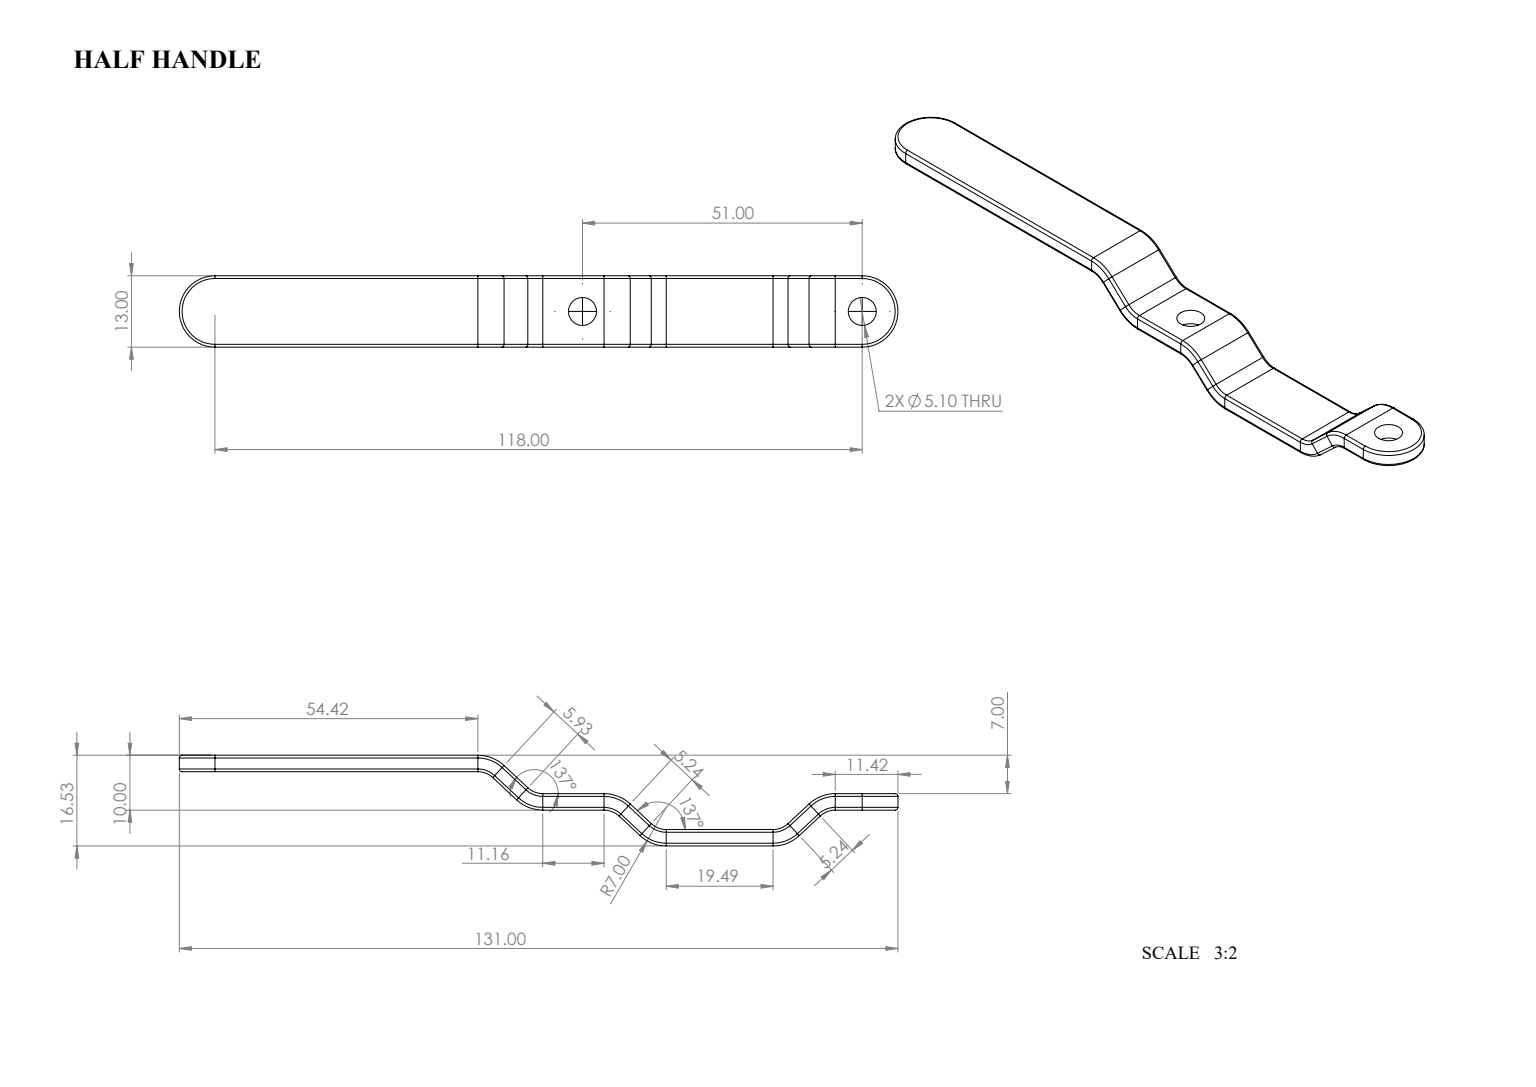
ISO-10303-21;
HEADER;
FILE_DESCRIPTION (('STEP AP214'),
    '1' );
FILE_NAME ('Half Handle.step',
    '2026-10-06T08:09:25',
    ( '' ),
    ( '' ),
    'SwSTEP 2.0',
    'SolidWorks 2021',
    '' );
FILE_SCHEMA (( 'AUTOMOTIVE_DESIGN' ));
ENDSEC;

DATA;
#3=ORIENTED_EDGE ( 'NONE', *, *, #3053, .T. ) ;
#15=CYLINDRICAL_SURFACE ( 'NONE', #19275, 7.000000000000075495 ) ;
#16=FACE_OUTER_BOUND ( 'NONE', #19834, .T. ) ;
#35=ORIENTED_EDGE ( 'NONE', *, *, #12081, .T. ) ;
#44=EDGE_CURVE ( 'NONE', #15578, #10139, #5040, .T. ) ;
#57=TOROIDAL_SURFACE ( 'NONE', #21466, 6.000000000000000000, 0.5000000000000000000 ) ;
#61=ORIENTED_EDGE ( 'NONE', *, *, #623, .T. ) ;
#71=DIRECTION ( 'NONE',  ( -1.000000000000000000, -5.598259082250514647E-17, -3.330669073875432643E-16 ) ) ;
#74=CARTESIAN_POINT ( 'NONE',  ( 119.5756419024615838, -4.500000000000059508, -6.499999999999970690 ) ) ;
#75=AXIS2_PLACEMENT_3D ( 'NONE', #705, #21992, #9988 ) ;
#79=CARTESIAN_POINT ( 'NONE',  ( 2.775557561562891351E-14, 0.000000000000000000, -6.000000000000019540 ) ) ;
#87=ORIENTED_EDGE ( 'NONE', *, *, #1268, .T. ) ;
#102=DIRECTION ( 'NONE',  ( 0.000000000000000000, 0.000000000000000000, 1.000000000000000000 ) ) ;
#108=EDGE_CURVE ( 'NONE', #6044, #8580, #6954, .T. ) ;
#110=DIRECTION ( 'NONE',  ( 3.032184104443271834E-30, 1.000000000000000000, 4.437342591868167759E-31 ) ) ;
#113=DIRECTION ( 'NONE',  ( -0.7313537016191756779, 0.6819983600624930364, -4.478224685260177339E-16 ) ) ;
#125=DIRECTION ( 'NONE',  ( -3.885780586188016830E-16, -4.437342591868156373E-31, 1.000000000000000000 ) ) ;
#147=ORIENTED_EDGE ( 'NONE', *, *, #4920, .T. ) ;
#148=CARTESIAN_POINT ( 'NONE',  ( 119.5756419024615269, -11.00000000000006573, 6.000000000000081712 ) ) ;
#165=FACE_OUTER_BOUND ( 'NONE', #636, .T. ) ;
#169=ADVANCED_FACE ( 'NONE', ( #20745 ), #4609, .T. ) ;
#179=LINE ( 'NONE', #15827, #9133 ) ;
#210=LINE ( 'NONE', #7721, #18126 ) ;
#216=DIRECTION ( 'NONE',  ( 1.000000000000000000, 5.598259082250514647E-17, 3.330669073875432643E-16 ) ) ;
#231=CARTESIAN_POINT ( 'NONE',  ( 54.42435809754113052, -4.000000000000003553, -6.000000000000012434 ) ) ;
#232=LINE ( 'NONE', #4899, #1007 ) ;
#234=DIRECTION ( 'NONE',  ( 0.000000000000000000, 0.000000000000000000, 1.000000000000000000 ) ) ;
#239=DIRECTION ( 'NONE',  ( -1.000000000000000000, 0.000000000000000000, -3.330669073875408978E-16 ) ) ;
#246=ORIENTED_EDGE ( 'NONE', *, *, #14573, .F. ) ;
#248=ADVANCED_FACE ( 'NONE', ( #1437 ), #12950, .T. ) ;
#253=ADVANCED_FACE ( 'NONE', ( #8611 ), #5204, .T. ) ;
#262=LINE ( 'NONE', #18378, #17735 ) ;
#265=CIRCLE ( 'NONE', #18661, 4.500000000000045297 ) ;
#271=ORIENTED_EDGE ( 'NONE', *, *, #15321, .T. ) ;
#273=VERTEX_POINT ( 'NONE', #8728 ) ;
#277=EDGE_LOOP ( 'NONE', ( #6331, #5519, #19401, #7762 ) ) ;
#284=ORIENTED_EDGE ( 'NONE', *, *, #7716, .T. ) ;
#287=CARTESIAN_POINT ( 'NONE',  ( 54.42435809754115894, 2.999999999999947153, 6.000000000000136779 ) ) ;
#291=LINE ( 'NONE', #18180, #3856 ) ;
#299=AXIS2_PLACEMENT_3D ( 'NONE', #21279, #216, #10679 ) ;
#306=EDGE_LOOP ( 'NONE', ( #6785, #17565, #11984, #16573 ) ) ;
#314=ORIENTED_EDGE ( 'NONE', *, *, #20628, .F. ) ;
#315=CARTESIAN_POINT ( 'NONE',  ( 56.34099918003215635, 0.3656768508095153969, -5.999999999999991118 ) ) ;
#317=FACE_OUTER_BOUND ( 'NONE', #6393, .T. ) ;
#324=CARTESIAN_POINT ( 'NONE',  ( 88.75737332930587797, -10.52760560296347947, 6.500000000000075495 ) ) ;
#330=AXIS2_PLACEMENT_3D ( 'NONE', #11225, #18403, #21944 ) ;
#345=VECTOR ( 'NONE', #22191, 1000.000000000000114 ) ;
#349=CARTESIAN_POINT ( 'NONE',  ( 66.26395429947835680, -6.500000000000005329, -6.500000000000081712 ) ) ;
#350=FACE_OUTER_BOUND ( 'NONE', #12361, .T. ) ;
#351=DIRECTION ( 'NONE',  ( -1.000000000000000000, -2.699383410053119644E-30, -3.330669073875432643E-16 ) ) ;
#354=FACE_OUTER_BOUND ( 'NONE', #13443, .T. ) ;
#355=LINE ( 'NONE', #4202, #16056 ) ;
#362=FACE_OUTER_BOUND ( 'NONE', #15798, .T. ) ;
#374=EDGE_LOOP ( 'NONE', ( #13092, #17364, #11552, #11898 ) ) ;
#375=CARTESIAN_POINT ( 'NONE',  ( 108.2426266706972058, -6.527605602963671316, -6.500000000000019540 ) ) ;
#386=AXIS2_PLACEMENT_3D ( 'NONE', #9346, #14745, #22046 ) ;
#397=ORIENTED_EDGE ( 'NONE', *, *, #3887, .T. ) ;
#402=ORIENTED_EDGE ( 'NONE', *, *, #7849, .T. ) ;
#417=ORIENTED_EDGE ( 'NONE', *, *, #17478, .T. ) ;
#430=VECTOR ( 'NONE', #5625, 1000.000000000000114 ) ;
#447=ORIENTED_EDGE ( 'NONE', *, *, #16080, .F. ) ;
#450=DIRECTION ( 'NONE',  ( 3.032184104443272185E-30, 1.000000000000000000, -7.395570986447005381E-32 ) ) ;
#457=DIRECTION ( 'NONE',  ( -3.885780586188016830E-16, -4.437342591868156373E-31, 1.000000000000000000 ) ) ;
#467=CARTESIAN_POINT ( 'NONE',  ( 61.83096495907209089, -4.753799060524588782, 6.500000000000179412 ) ) ;
#468=CARTESIAN_POINT ( 'NONE',  ( 108.2426266706970353, -6.527605602963587828, 6.500000000000199840 ) ) ;
#504=CIRCLE ( 'NONE', #11000, 0.5000000000000033307 ) ;
#519=EDGE_CURVE ( 'NONE', #5606, #14358, #3300, .T. ) ;
#522=VERTEX_POINT ( 'NONE', #22826 ) ;
#542=DIRECTION ( 'NONE',  ( -4.003208021484906984E-16, 0.000000000000000000, 1.000000000000000000 ) ) ;
#550=DIRECTION ( 'NONE',  ( -1.000000000000000000, 7.477632011778292156E-48, -3.885780586188017323E-16 ) ) ;
#552=CLOSED_SHELL ( 'NONE', ( #5998, #12224, #22308, #16919, #14838, #610, #17542, #5814, #9022, #13526, #11262, #22008, #12800, #12847, #7373, #1350, #6364, #15263, #7801, #12373, #8928, #19017, #2140, #3076, #20370, #13608, #253, #7841, #18717, #10097, #22749, #10522, #2281, #5956, #13001, #8303, #15121, #2768, #13653, #19566, #15676, #20490, #22930, #18573, #22774, #6659, #16164, #8294, #8684, #5013, #2022, #6644, #17118, #6392, #7909, #19774, #10655, #21216, #20630, #3506, #12830, #8059, #21456, #15577, #6060, #7869, #10599, #15845, #17708, #12378, #6678, #19804, #5540, #19247, #5780, #21642, #16295, #19370, #13968, #12259, #9663, #1243, #17730, #12097, #1896, #687, #20297, #21117, #20746, #4689, #12071, #17436, #7470, #15967, #6389, #3205, #13846, #14982, #16297, #15524, #6855, #17451, #21619, #3605, #12668, #248, #4912, #22621, #14523, #15294, #7422, #169, #14422, #14548 ) ) ;
#568=SHAPE_REPRESENTATION_RELATIONSHIP ( 'NONE' , 'NONE' ,  #15574, #22653 ) ;
#572=EDGE_LOOP ( 'NONE', ( #5727, #7824, #20773, #18885 ) ) ;
#573=CARTESIAN_POINT ( 'NONE',  ( 115.1426525620552894, -6.246200939475421876, 6.000000000000158096 ) ) ;
#585=CARTESIAN_POINT ( 'NONE',  ( 58.85734743794737511, 0.7537990605245015185, -6.499999999999895195 ) ) ;
#589=DIRECTION ( 'NONE',  ( 0.6819983600624954789, 0.7313537016191733464, 7.771699578536739269E-16 ) ) ;
#590=CARTESIAN_POINT ( 'NONE',  ( 66.26395429947839943, -7.000000000000006217, -6.499999999999999112 ) ) ;
#593=VECTOR ( 'NONE', #7277, 1000.000000000000000 ) ;
#601=DIRECTION ( 'NONE',  ( -1.000000000000000000, -2.699383410053119644E-30, -3.330669073875432643E-16 ) ) ;
#610=ADVANCED_FACE ( 'NONE', ( #4927 ), #12094, .F. ) ;
#623=EDGE_CURVE ( 'NONE', #15916, #8376, #10912, .T. ) ;
#626=EDGE_CURVE ( 'NONE', #2822, #21618, #7403, .T. ) ;
#636=EDGE_LOOP ( 'NONE', ( #3298, #20514, #22207, #18614 ) ) ;
#669=DIRECTION ( 'NONE',  ( 1.000000000000000000, 2.699383410053119644E-30, 3.330669073875432643E-16 ) ) ;
#677=DIRECTION ( 'NONE',  ( 3.032184104443272185E-30, 1.000000000000000000, -7.395570986447005381E-32 ) ) ;
#678=AXIS2_PLACEMENT_3D ( 'NONE', #13630, #15379, #15731 ) ;
#683=SURFACE_SIDE_STYLE ('',( #9387 ) ) ;
#687=ADVANCED_FACE ( 'NONE', ( #21534 ), #20120, .T. ) ;
#693=DIRECTION ( 'NONE',  ( 0.6819983600624958120, 0.7313537016191731244, 7.771699578536736311E-16 ) ) ;
#694=LINE ( 'NONE', #5870, #6828 ) ;
#700=VERTEX_POINT ( 'NONE', #19396 ) ;
#701=LINE ( 'NONE', #13282, #21174 ) ;
#704=ORIENTED_EDGE ( 'NONE', *, *, #6611, .T. ) ;
#705=CARTESIAN_POINT ( 'NONE',  ( 54.42435809754115894, 2.499999999999946709, 6.000000000000136779 ) ) ;
#712=( GEOMETRIC_REPRESENTATION_CONTEXT ( 3 ) GLOBAL_UNCERTAINTY_ASSIGNED_CONTEXT ( ( #16830 ) ) GLOBAL_UNIT_ASSIGNED_CONTEXT ( ( #5192, #21975, #2204 ) ) REPRESENTATION_CONTEXT ( 'NONE', 'WORKASPACE' ) );
#717=ORIENTED_EDGE ( 'NONE', *, *, #22216, .T. ) ;
#720=DIRECTION ( 'NONE',  ( 1.000000000000000000, 2.699383410053119644E-30, 3.330669073875432643E-16 ) ) ;
#730=AXIS2_PLACEMENT_3D ( 'NONE', #8897, #17709, #6781 ) ;
#740=EDGE_LOOP ( 'NONE', ( #2269, #18796, #14103, #12386 ) ) ;
#746=VERTEX_POINT ( 'NONE', #5056 ) ;
#763=LINE ( 'NONE', #20873, #11220 ) ;
#766=EDGE_CURVE ( 'NONE', #11435, #5256, #21184, .T. ) ;
#773=CIRCLE ( 'NONE', #10164, 0.5000000000000038858 ) ;
#788=EDGE_CURVE ( 'NONE', #15578, #6044, #1862, .T. ) ;
#795=CARTESIAN_POINT ( 'NONE',  ( 6.500000000000227374, 2.500000000000196287, 6.000000000000213163 ) ) ;
#797=FILL_AREA_STYLE ('',( #2314 ) ) ;
#801=ORIENTED_EDGE ( 'NONE', *, *, #10616, .F. ) ;
#802=AXIS2_PLACEMENT_3D ( 'NONE', #12809, #5296, #239 ) ;
#816=CARTESIAN_POINT ( 'NONE',  ( 6.500000000000366818, 2.500000000000196287, 6.500000000000123457 ) ) ;
#821=AXIS2_PLACEMENT_3D ( 'NONE', #3851, #21982, #16435 ) ;
#831=CIRCLE ( 'NONE', #9848, 4.000000000000045297 ) ;
#843=DIRECTION ( 'NONE',  ( 1.000000000000000000, 0.000000000000000000, 4.336808689941968432E-16 ) ) ;
#861=ORIENTED_EDGE ( 'NONE', *, *, #20330, .T. ) ;
#868=CARTESIAN_POINT ( 'NONE',  ( 88.75737332930597745, -13.52760560296348302, 6.500000000000103029 ) ) ;
#934=DIRECTION ( 'NONE',  ( 0.000000000000000000, 0.000000000000000000, 1.000000000000000000 ) ) ;
#935=DIRECTION ( 'NONE',  ( -0.7313537016191756779, 0.6819983600624930364, -4.478224685260177339E-16 ) ) ;
#941=DIRECTION ( 'NONE',  ( -1.000000000000000000, -2.699383410053119644E-30, -3.330669073875432643E-16 ) ) ;
#961=DIRECTION ( 'NONE',  ( -1.000000000000000000, -2.699383410053119644E-30, -3.330669073875432643E-16 ) ) ;
#973=DIRECTION ( 'NONE',  ( -1.000000000000000000, -2.699383410053119644E-30, -3.330669073875432643E-16 ) ) ;
#979=EDGE_CURVE ( 'NONE', #11432, #5256, #232, .T. ) ;
#982=ORIENTED_EDGE ( 'NONE', *, *, #6089, .T. ) ;
#1000=DIRECTION ( 'NONE',  ( 3.885780586188016830E-16, 4.437342591868156373E-31, -1.000000000000000000 ) ) ;
#1007=VECTOR ( 'NONE', #1279, 1000.000000000000000 ) ;
#1053=AXIS2_PLACEMENT_3D ( 'NONE', #9891, #961, #12100 ) ;
#1060=CARTESIAN_POINT ( 'NONE',  ( 119.5756419024615838, -6.500000000000061284, -5.999999999999984901 ) ) ;
#1064=LINE ( 'NONE', #10212, #4061 ) ;
#1070=AXIS2_PLACEMENT_3D ( 'NONE', #12709, #1992, #1876 ) ;
#1073=ORIENTED_EDGE ( 'NONE', *, *, #6663, .T. ) ;
#1075=CARTESIAN_POINT ( 'NONE',  ( 59.19834661797866460, 1.119475911334100182, 6.500000000000130562 ) ) ;
#1086=EDGE_CURVE ( 'NONE', #16898, #10112, #2677, .T. ) ;
#1091=AXIS2_PLACEMENT_3D ( 'NONE', #18092, #10900, #9266 ) ;
#1096=ORIENTED_EDGE ( 'NONE', *, *, #3338, .T. ) ;
#1106=CARTESIAN_POINT ( 'NONE',  ( 85.68838070902455684, -9.818697260249752645, 6.000000000000136779 ) ) ;
#1110=EDGE_CURVE ( 'NONE', #11343, #15739, #11136, .T. ) ;
#1111=DIRECTION ( 'NONE',  ( 3.032184104443272185E-30, 1.000000000000000000, -7.395570986447005381E-32 ) ) ;
#1116=DIRECTION ( 'NONE',  ( -0.7313537016191773432, 0.6819983600624913711, 1.628001950178159721E-16 ) ) ;
#1118=EDGE_CURVE ( 'NONE', #13735, #11435, #20927, .T. ) ;
#1122=DIRECTION ( 'NONE',  ( 3.885780586188016830E-16, 4.437342591868156373E-31, -1.000000000000000000 ) ) ;
#1126=EDGE_LOOP ( 'NONE', ( #14306, #4368, #8291, #9544 ) ) ;
#1128=ORIENTED_EDGE ( 'NONE', *, *, #17861, .F. ) ;
#1138=DIRECTION ( 'NONE',  ( -3.885780586188016830E-16, -4.437342591868156373E-31, 1.000000000000000000 ) ) ;
#1145=AXIS2_PLACEMENT_3D ( 'NONE', #5595, #16499, #9229 ) ;
#1156=ORIENTED_EDGE ( 'NONE', *, *, #626, .F. ) ;
#1157=ORIENTED_EDGE ( 'NONE', *, *, #788, .T. ) ;
#1159=DIRECTION ( 'NONE',  ( -0.6819983600625064701, -0.7313537016191632434, 0.000000000000000000 ) ) ;
#1160=ORIENTED_EDGE ( 'NONE', *, *, #10930, .T. ) ;
#1166=CARTESIAN_POINT ( 'NONE',  ( 113.0166151911346617, -11.64708151429780258, 6.500000000000110134 ) ) ;
#1170=DIRECTION ( 'NONE',  ( 1.000000000000000000, 2.699383410053119644E-30, 3.330669073875432643E-16 ) ) ;
#1173=EDGE_CURVE ( 'NONE', #746, #20880, #10395, .T. ) ;
#1210=EDGE_CURVE ( 'NONE', #23117, #22529, #21623, .T. ) ;
#1211=EDGE_LOOP ( 'NONE', ( #10687, #3, #21937, #717 ) ) ;
#1231=FACE_OUTER_BOUND ( 'NONE', #3457, .T. ) ;
#1243=ADVANCED_FACE ( 'NONE', ( #18852 ), #10767, .T. ) ;
#1244=CIRCLE ( 'NONE', #16614, 0.4999999999999997224 ) ;
#1253=DIRECTION ( 'NONE',  ( -0.7313537016191753448, -0.6819983600624934805, -1.628001950178158981E-16 ) ) ;
#1254=DIRECTION ( 'NONE',  ( 3.032184104443271834E-30, 1.000000000000000000, 4.437342591868167759E-31 ) ) ;
#1268=EDGE_CURVE ( 'NONE', #6421, #12056, #9925, .T. ) ;
#1269=EDGE_LOOP ( 'NONE', ( #6367, #10826, #1697, #13479 ) ) ;
#1271=EDGE_CURVE ( 'NONE', #11689, #5606, #19039, .T. ) ;
#1279=DIRECTION ( 'NONE',  ( -0.7313537016191735685, 0.6819983600624951459, -3.923113172947598083E-16 ) ) ;
#1288=DIRECTION ( 'NONE',  ( 0.000000000000000000, 0.000000000000000000, 1.000000000000000000 ) ) ;
#1294=AXIS2_PLACEMENT_3D ( 'NONE', #19329, #22516, #6859 ) ;
#1303=LINE ( 'NONE', #8350, #11618 ) ;
#1311=VECTOR ( 'NONE', #6045, 1000.000000000000114 ) ;
#1331=EDGE_LOOP ( 'NONE', ( #20654, #22644, #11760, #18194 ) ) ;
#1332=CARTESIAN_POINT ( 'NONE',  ( 88.75737332930594903, -6.527605602963476805, 6.500000000000151879 ) ) ;
#1335=CARTESIAN_POINT ( 'NONE',  ( 88.75737332930594903, -13.02760560296348302, 6.000000000000130562 ) ) ;
#1350=ADVANCED_FACE ( 'NONE', ( #7920 ), #4263, .T. ) ;
#1369=PLANE ( 'NONE',  #20431 ) ;
#1378=ORIENTED_EDGE ( 'NONE', *, *, #10707, .F. ) ;
#1389=CARTESIAN_POINT ( 'NONE',  ( 119.5756419024615838, -11.00000000000006573, -6.500000000000075495 ) ) ;
#1391=DIRECTION ( 'NONE',  ( 0.6819983600624981435, -0.7313537016191709039, 0.000000000000000000 ) ) ;
#1409=ORIENTED_EDGE ( 'NONE', *, *, #4321, .T. ) ;
#1421=DIRECTION ( 'NONE',  ( -3.885780586188016830E-16, -4.437342591868156373E-31, 1.000000000000000000 ) ) ;
#1427=ORIENTED_EDGE ( 'NONE', *, *, #5079, .T. ) ;
#1436=CARTESIAN_POINT ( 'NONE',  ( 58.85734743794750301, 0.7537990605245015185, -5.999999999999880096 ) ) ;
#1437=FACE_OUTER_BOUND ( 'NONE', #5827, .T. ) ;
#1440=CARTESIAN_POINT ( 'NONE',  ( 80.49335071782263640, -7.708908342713538531, 6.500000000000033751 ) ) ;
#1453=DIRECTION ( 'NONE',  ( 3.885780586188016830E-16, 4.437342591868156373E-31, -1.000000000000000000 ) ) ;
#1457=ORIENTED_EDGE ( 'NONE', *, *, #11127, .F. ) ;
#1469=ORIENTED_EDGE ( 'NONE', *, *, #108, .F. ) ;
#1474=PLANE ( 'NONE',  #8000 ) ;
#1495=VERTEX_POINT ( 'NONE', #1440 ) ;
#1511=DIRECTION ( 'NONE',  ( 0.7313537016191745677, 0.6819983600624940356, 1.072890437865584285E-16 ) ) ;
#1518=ORIENTED_EDGE ( 'NONE', *, *, #20201, .T. ) ;
#1522=EDGE_CURVE ( 'NONE', #22506, #18271, #8616, .T. ) ;
#1528=EDGE_CURVE ( 'NONE', #11543, #15515, #17880, .T. ) ;
#1529=DIRECTION ( 'NONE',  ( 0.6819983600625074693, -0.7313537016191621332, 1.110084618464482116E-16 ) ) ;
#1549=CIRCLE ( 'NONE', #7564, 0.5000000000000038858 ) ;
#1553=CARTESIAN_POINT ( 'NONE',  ( 82.19834661797897013, -5.880524088665628923, 6.500000000000151879 ) ) ;
#1566=AXIS2_PLACEMENT_3D ( 'NONE', #17345, #1253, #8430 ) ;
#1567=DIRECTION ( 'NONE',  ( 3.885780586188016830E-16, 4.437342591868156373E-31, -1.000000000000000000 ) ) ;
#1568=PLANE ( 'NONE',  #3642 ) ;
#1573=ORIENTED_EDGE ( 'NONE', *, *, #2157, .F. ) ;
#1578=AXIS2_PLACEMENT_3D ( 'NONE', #16932, #6256, #843 ) ;
#1587=CARTESIAN_POINT ( 'NONE',  ( 77.42435809754145737, -6.499999999999811706, -6.499999999999984901 ) ) ;
#1604=CIRCLE ( 'NONE', #3842, 0.5000000000000038858 ) ;
#1609=PRODUCT_DEFINITION_SHAPE ( 'NONE', 'NONE',  #17672 ) ;
#1610=ORIENTED_EDGE ( 'NONE', *, *, #10575, .T. ) ;
#1611=CARTESIAN_POINT ( 'NONE',  ( 80.15235153779146060, -8.074585193523137860, 6.000000000000109246 ) ) ;
#1614=CARTESIAN_POINT ( 'NONE',  ( 77.42435809754135789, -10.99999999999981526, 6.500000000000123457 ) ) ;
#1617=LINE ( 'NONE', #19377, #10224 ) ;
#1621=VECTOR ( 'NONE', #16837, 1000.000000000000000 ) ;
#1634=AXIS2_PLACEMENT_3D ( 'NONE', #16389, #23134, #5714 ) ;
#1660=AXIS2_PLACEMENT_3D ( 'NONE', #8212, #6447, #1159 ) ;
#1667=EDGE_LOOP ( 'NONE', ( #61, #23206, #12396, #397 ) ) ;
#1668=ORIENTED_EDGE ( 'NONE', *, *, #16268, .F. ) ;
#1676=DIRECTION ( 'NONE',  ( -3.241725282392603095E-30, -1.000000000000000000, 2.218671295934100958E-31 ) ) ;
#1697=ORIENTED_EDGE ( 'NONE', *, *, #2183, .F. ) ;
#1701=EDGE_LOOP ( 'NONE', ( #3380, #9857, #18964, #1457 ) ) ;
#1709=DIRECTION ( 'NONE',  ( 3.330669073875432643E-16, 4.437342591868153746E-31, -1.000000000000000000 ) ) ;
#1723=EDGE_CURVE ( 'NONE', #19565, #9737, #4469, .T. ) ;
#1724=CARTESIAN_POINT ( 'NONE',  ( 73.50000000000116529, -13.52760560296348302, 3.469446951953614189E-14 ) ) ;
#1739=CYLINDRICAL_SURFACE ( 'NONE', #10098, 0.4999999999999978351 ) ;
#1758=AXIS2_PLACEMENT_3D ( 'NONE', #10952, #18261, #3785 ) ;
#1769=VECTOR ( 'NONE', #973, 1000.000000000000000 ) ;
#1795=DIRECTION ( 'NONE',  ( 0.000000000000000000, 0.000000000000000000, 1.000000000000000000 ) ) ;
#1798=DIRECTION ( 'NONE',  ( -0.7313537016191746787, -0.6819983600624940356, -1.072890437865584285E-16 ) ) ;
#1799=DIRECTION ( 'NONE',  ( 3.885780586188016830E-16, 4.437342591868156373E-31, -1.000000000000000000 ) ) ;
#1812=ORIENTED_EDGE ( 'NONE', *, *, #16958, .F. ) ;
#1814=AXIS2_PLACEMENT_3D ( 'NONE', #21549, #12588, #18016 ) ;
#1821=LINE ( 'NONE', #23253, #8978 ) ;
#1822=CARTESIAN_POINT ( 'NONE',  ( 73.50000000000116529, -6.999999999999811706, -2.549999999999999822 ) ) ;
#1827=ORIENTED_EDGE ( 'NONE', *, *, #20596, .F. ) ;
#1828=CIRCLE ( 'NONE', #22491, 0.5000000000000038858 ) ;
#1829=DIRECTION ( 'NONE',  ( 3.885780586188016830E-16, 4.437342591868156373E-31, -1.000000000000000000 ) ) ;
#1839=CYLINDRICAL_SURFACE ( 'NONE', #20758, 4.000000000000045297 ) ;
#1860=AXIS2_PLACEMENT_3D ( 'NONE', #19707, #7012, #12163 ) ;
#1862=LINE ( 'NONE', #9046, #20910 ) ;
#1865=ORIENTED_EDGE ( 'NONE', *, *, #2806, .F. ) ;
#1871=DIRECTION ( 'NONE',  ( 1.000000000000000000, 2.699383410053119644E-30, 3.330669073875432643E-16 ) ) ;
#1876=DIRECTION ( 'NONE',  ( 0.000000000000000000, 0.000000000000000000, 1.000000000000000000 ) ) ;
#1889=VECTOR ( 'NONE', #3441, 1000.000000000000000 ) ;
#1892=EDGE_CURVE ( 'NONE', #4169, #16118, #8245, .T. ) ;
#1894=FACE_OUTER_BOUND ( 'NONE', #9998, .T. ) ;
#1896=ADVANCED_FACE ( 'NONE', ( #22591 ), #19404, .T. ) ;
#1908=AXIS2_PLACEMENT_3D ( 'NONE', #16553, #16096, #10814 ) ;
#1909=AXIS2_PLACEMENT_3D ( 'NONE', #12173, #5123, #19476 ) ;
#1912=EDGE_CURVE ( 'NONE', #22610, #5349, #17519, .T. ) ;
#1918=ORIENTED_EDGE ( 'NONE', *, *, #12888, .F. ) ;
#1920=DIRECTION ( 'NONE',  ( 1.000000000000000000, 2.699383410053119644E-30, 3.330669073875432643E-16 ) ) ;
#1928=DIRECTION ( 'NONE',  ( -1.000000000000000000, -2.699383410053119644E-30, -3.330669073875432643E-16 ) ) ;
#1929=CARTESIAN_POINT ( 'NONE',  ( 54.42435809754115894, 0.4999999999999449329, -5.999999999999950262 ) ) ;
#1934=ORIENTED_EDGE ( 'NONE', *, *, #20891, .F. ) ;
#1946=FACE_OUTER_BOUND ( 'NONE', #3552, .T. ) ;
#1947=CARTESIAN_POINT ( 'NONE',  ( 108.2426266706970353, -6.527605602963587828, 6.500000000000199840 ) ) ;
#1949=DIRECTION ( 'NONE',  ( 3.885780586188016830E-16, 4.437342591868156373E-31, -1.000000000000000000 ) ) ;
#1950=CIRCLE ( 'NONE', #6480, 6.500000000000075495 ) ;
#1955=CIRCLE ( 'NONE', #8719, 6.500000000000075495 ) ;
#1956=CARTESIAN_POINT ( 'NONE',  ( 88.75737332930596324, -13.52760560296348302, -6.499999999999964473 ) ) ;
#1967=CIRCLE ( 'NONE', #15113, 0.5000000000000038858 ) ;
#1968=ORIENTED_EDGE ( 'NONE', *, *, #20201, .F. ) ;
#1983=CARTESIAN_POINT ( 'NONE',  ( 119.5756419024615553, -11.00000000000006573, 6.500000000000012434 ) ) ;
#1992=DIRECTION ( 'NONE',  ( -1.000000000000000000, -2.699383410053119644E-30, -3.330669073875432643E-16 ) ) ;
#2004=DIRECTION ( 'NONE',  ( -1.000000000000000000, 1.773272886554051558E-14, -3.854941057726199147E-16 ) ) ;
#2015=DIRECTION ( 'NONE',  ( -1.000000000000000000, 1.847414967615758933E-47, -3.885780586188017323E-16 ) ) ;
#2022=ADVANCED_FACE ( 'NONE', ( #16 ), #14344, .T. ) ;
#2040=EDGE_CURVE ( 'NONE', #10112, #11689, #17882, .T. ) ;
#2042=DIRECTION ( 'NONE',  ( -1.000000000000000000, -2.699383410053119644E-30, -3.330669073875432643E-16 ) ) ;
#2062=EDGE_CURVE ( 'NONE', #15653, #23176, #8567, .T. ) ;
#2078=CARTESIAN_POINT ( 'NONE',  ( 61.48996577904087957, -5.119475911334187224, -5.999999999999943157 ) ) ;
#2091=DIRECTION ( 'NONE',  ( -1.000000000000000000, 0.000000000000000000, -4.336808689941968432E-16 ) ) ;
#2106=CARTESIAN_POINT ( 'NONE',  ( 86.02937988905577527, -11.02760560296348125, -5.999999999999991118 ) ) ;
#2115=ORIENTED_EDGE ( 'NONE', *, *, #17411, .T. ) ;
#2129=LINE ( 'NONE', #14497, #20800 ) ;
#2140=ADVANCED_FACE ( 'NONE', ( #16905 ), #2223, .T. ) ;
#2142=ORIENTED_EDGE ( 'NONE', *, *, #9809, .F. ) ;
#2145=ORIENTED_EDGE ( 'NONE', *, *, #12997, .F. ) ;
#2155=CARTESIAN_POINT ( 'NONE',  ( 110.9706201109470811, -9.453020409440348715, -5.999999999999956479 ) ) ;
#2157=EDGE_CURVE ( 'NONE', #746, #9743, #355, .T. ) ;
#2165=DIRECTION ( 'NONE',  ( 0.000000000000000000, 0.000000000000000000, 1.000000000000000000 ) ) ;
#2171=AXIS2_PLACEMENT_3D ( 'NONE', #12179, #17600, #23264 ) ;
#2172=EDGE_LOOP ( 'NONE', ( #20562, #16691, #3291, #6613 ) ) ;
#2174=FACE_OUTER_BOUND ( 'NONE', #14632, .T. ) ;
#2178=ORIENTED_EDGE ( 'NONE', *, *, #5139, .F. ) ;
#2183=EDGE_CURVE ( 'NONE', #522, #22680, #12297, .T. ) ;
#2188=DIRECTION ( 'NONE',  ( 1.000000000000000000, 1.599800538956372742E-14, 3.854941057726199147E-16 ) ) ;
#2197=CYLINDRICAL_SURFACE ( 'NONE', #13937, 7.000000000000075495 ) ;
#2204=( NAMED_UNIT ( * ) SI_UNIT ( $, .STERADIAN. ) SOLID_ANGLE_UNIT ( ) );
#2209=EDGE_CURVE ( 'NONE', #18644, #14732, #20963, .T. ) ;
#2213=DIRECTION ( 'NONE',  ( -0.7313537016191794526, -0.6819983600624889286, -4.403559511741029625E-16 ) ) ;
#2215=ORIENTED_EDGE ( 'NONE', *, *, #1528, .T. ) ;
#2223=PLANE ( 'NONE',  #22844 ) ;
#2226=CARTESIAN_POINT ( 'NONE',  ( 77.42435809754137210, -6.999999999999811706, 6.500000000000081712 ) ) ;
#2230=PLANE ( 'NONE',  #10685 ) ;
#2231=CARTESIAN_POINT ( 'NONE',  ( 119.9981234580896796, -4.453056000818161664, 6.000000000000123457 ) ) ;
#2235=EDGE_CURVE ( 'NONE', #19565, #12056, #7444, .T. ) ;
#2252=DIRECTION ( 'NONE',  ( -0.6819983600624998088, -0.7313537016191693496, 0.000000000000000000 ) ) ;
#2253=DIRECTION ( 'NONE',  ( 3.241725282392603095E-30, 1.000000000000000000, -2.218671295934100958E-31 ) ) ;
#2256=FILL_AREA_STYLE_COLOUR ( '', #4776 ) ;
#2261=EDGE_CURVE ( 'NONE', #4634, #9218, #7087, .T. ) ;
#2265=ORIENTED_EDGE ( 'NONE', *, *, #12537, .T. ) ;
#2269=ORIENTED_EDGE ( 'NONE', *, *, #8952, .T. ) ;
#2273=EDGE_LOOP ( 'NONE', ( #2521, #9741, #12678, #4333 ) ) ;
#2274=ORIENTED_EDGE ( 'NONE', *, *, #13394, .T. ) ;
#2281=ADVANCED_FACE ( 'NONE', ( #22568 ), #4903, .T. ) ;
#2297=CIRCLE ( 'NONE', #75, 0.5000000000000038858 ) ;
#2298=VECTOR ( 'NONE', #19851, 1000.000000000000000 ) ;
#2314=FILL_AREA_STYLE_COLOUR ( '', #14588 ) ;
#2331=CARTESIAN_POINT ( 'NONE',  ( 108.2426266706970779, -6.527605602963587828, 6.000000000000109246 ) ) ;
#2332=AXIS2_PLACEMENT_3D ( 'NONE', #5854, #16756, #9373 ) ;
#2336=CARTESIAN_POINT ( 'NONE',  ( 109.3164911904586916, -11.67918431276163105, -6.000000000000060396 ) ) ;
#2344=CARTESIAN_POINT ( 'NONE',  ( 116.8476484622115805, -8.074585193523331483, -5.999999999999956479 ) ) ;
#2369=CARTESIAN_POINT ( 'NONE',  ( 57.49335071782248008, -0.7089083427137543580, 6.500000000000088818 ) ) ;
#2381=AXIS2_PLACEMENT_3D ( 'NONE', #1956, #9154, #16314 ) ;
#2386=EDGE_LOOP ( 'NONE', ( #18996, #18444, #16291, #5485 ) ) ;
#2389=AXIS2_PLACEMENT_3D ( 'NONE', #22561, #4553, #2801 ) ;
#2405=AXIS2_PLACEMENT_3D ( 'NONE', #5125, #12286, #12409 ) ;
#2416=DIRECTION ( 'NONE',  ( -0.7313537016191734574, 0.6819983600624954789, -3.733258675956565293E-18 ) ) ;
#2419=CIRCLE ( 'NONE', #9935, 0.5000000000000038858 ) ;
#2435=CARTESIAN_POINT ( 'NONE',  ( 108.2426266706970637, -11.02760560296359138, 5.999999999999984901 ) ) ;
#2451=DIRECTION ( 'NONE',  ( -3.885780586188016830E-16, -4.437342591868156373E-31, 1.000000000000000000 ) ) ;
#2458=DIRECTION ( 'NONE',  ( 3.885780586188016830E-16, 4.437342591868156373E-31, -1.000000000000000000 ) ) ;
#2462=ORIENTED_EDGE ( 'NONE', *, *, #21922, .T. ) ;
#2464=ORIENTED_EDGE ( 'NONE', *, *, #5341, .T. ) ;
#2481=CARTESIAN_POINT ( 'NONE',  ( 124.5000000000019469, -6.500000000000061284, 4.857225732735059864E-14 ) ) ;
#2484=EDGE_CURVE ( 'NONE', #15515, #7123, #21845, .T. ) ;
#2486=LINE ( 'NONE', #20503, #13438 ) ;
#2487=CARTESIAN_POINT ( 'NONE',  ( 66.26395429947835680, -4.500000000000003553, -6.500000000000081712 ) ) ;
#2489=ORIENTED_EDGE ( 'NONE', *, *, #5645, .F. ) ;
#2490=TOROIDAL_SURFACE ( 'NONE', #8901, 6.500000000000000888, 0.5000000000000000000 ) ;
#2492=EDGE_LOOP ( 'NONE', ( #35, #15607, #5667, #17989 ) ) ;
#2493=UNCERTAINTY_MEASURE_WITH_UNIT (LENGTH_MEASURE( 1.000000000000000082E-05 ), #11423, 'distance_accuracy_value', 'NONE');
#2521=ORIENTED_EDGE ( 'NONE', *, *, #13323, .T. ) ;
#2525=CIRCLE ( 'NONE', #7048, 0.4999999999999984457 ) ;
#2531=DIRECTION ( 'NONE',  ( 0.6819983600624981435, -0.7313537016191709039, 0.000000000000000000 ) ) ;
#2538=AXIS2_PLACEMENT_3D ( 'NONE', #2743, #18987, #23079 ) ;
#2552=ORIENTED_EDGE ( 'NONE', *, *, #13276, .T. ) ;
#2567=DIRECTION ( 'NONE',  ( -1.000000000000000000, -2.699383410053119644E-30, -3.330669073875432643E-16 ) ) ;
#2572=DIRECTION ( 'NONE',  ( -3.032184104443272185E-30, -1.000000000000000000, 7.395570986447005381E-32 ) ) ;
#2576=CYLINDRICAL_SURFACE ( 'NONE', #6610, 0.5000000000000038858 ) ;
#2582=CIRCLE ( 'NONE', #19501, 4.000000000000045297 ) ;
#2593=EDGE_CURVE ( 'NONE', #16059, #19782, #2582, .T. ) ;
#2595=AXIS2_PLACEMENT_3D ( 'NONE', #10540, #18195, #9242 ) ;
#2610=ORIENTED_EDGE ( 'NONE', *, *, #15468, .F. ) ;
#2621=CARTESIAN_POINT ( 'NONE',  ( 119.5756419024614559, 2.499999999999974243, -5.999999999999963585 ) ) ;
#2628=APPLICATION_CONTEXT ( 'automotive_design' ) ;
#2639=CYLINDRICAL_SURFACE ( 'NONE', #9314, 7.000000000000075495 ) ;
#2640=EDGE_CURVE ( 'NONE', #23176, #18021, #6653, .T. ) ;
#2641=ORIENTED_EDGE ( 'NONE', *, *, #10946, .T. ) ;
#2643=EDGE_LOOP ( 'NONE', ( #9016, #7011, #20838, #17686 ) ) ;
#2653=CYLINDRICAL_SURFACE ( 'NONE', #7597, 0.4999999999999987232 ) ;
#2659=CARTESIAN_POINT ( 'NONE',  ( 119.5756419024615411, -7.000000000000006217, 6.000000000000095923 ) ) ;
#2665=EDGE_LOOP ( 'NONE', ( #9213, #15572, #3033, #14858 ) ) ;
#2673=DIRECTION ( 'NONE',  ( -0.7313537016191730133, 0.6819983600624957010, -5.924440990721418971E-17 ) ) ;
#2677=LINE ( 'NONE', #11614, #7400 ) ;
#2684=FACE_OUTER_BOUND ( 'NONE', #22293, .T. ) ;
#2688=CARTESIAN_POINT ( 'NONE',  ( 80.49335071782266482, -7.708908342713566064, -6.500000000000047073 ) ) ;
#2697=AXIS2_PLACEMENT_3D ( 'NONE', #18422, #11347, #18538 ) ;
#2705=FACE_OUTER_BOUND ( 'NONE', #15944, .T. ) ;
#2717=CIRCLE ( 'NONE', #5358, 6.000000000000047962 ) ;
#2721=ORIENTED_EDGE ( 'NONE', *, *, #5530, .F. ) ;
#2724=ORIENTED_EDGE ( 'NONE', *, *, #14425, .F. ) ;
#2726=ORIENTED_EDGE ( 'NONE', *, *, #22779, .F. ) ;
#2728=ORIENTED_EDGE ( 'NONE', *, *, #8529, .T. ) ;
#2734=DIRECTION ( 'NONE',  ( -1.000000000000000000, 1.847414967615758933E-47, -3.885780586188017323E-16 ) ) ;
#2737=DIRECTION ( 'NONE',  ( 0.000000000000000000, 0.000000000000000000, -1.000000000000000000 ) ) ;
#2743=CARTESIAN_POINT ( 'NONE',  ( 108.2426266706970637, -13.52760560296348302, 6.500000000000019540 ) ) ;
#2765=APPLICATION_CONTEXT ( 'automotive_design' ) ;
#2766=ORIENTED_EDGE ( 'NONE', *, *, #21500, .T. ) ;
#2768=ADVANCED_FACE ( 'NONE', ( #6428 ), #15115, .T. ) ;
#2786=EDGE_CURVE ( 'NONE', #17843, #3270, #1821, .T. ) ;
#2787=ORIENTED_EDGE ( 'NONE', *, *, #9230, .T. ) ;
#2792=ORIENTED_EDGE ( 'NONE', *, *, #16542, .T. ) ;
#2796=ORIENTED_EDGE ( 'NONE', *, *, #44, .T. ) ;
#2801=DIRECTION ( 'NONE',  ( 1.000000000000000000, -7.477632011778619108E-48, 3.885780586188017323E-16 ) ) ;
#2804=DIRECTION ( 'NONE',  ( -1.000000000000000000, -2.699383410053119644E-30, -3.330669073875432643E-16 ) ) ;
#2806=EDGE_CURVE ( 'NONE', #700, #9743, #12332, .T. ) ;
#2816=AXIS2_PLACEMENT_3D ( 'NONE', #19426, #3327, #12013 ) ;
#2817=LINE ( 'NONE', #2688, #3872 ) ;
#2821=ORIENTED_EDGE ( 'NONE', *, *, #2786, .F. ) ;
#2822=VERTEX_POINT ( 'NONE', #1587 ) ;
#2826=VERTEX_POINT ( 'NONE', #74 ) ;
#2829=EDGE_CURVE ( 'NONE', #6497, #19367, #17467, .T. ) ;
#2845=ORIENTED_EDGE ( 'NONE', *, *, #6203, .F. ) ;
#2853=EDGE_LOOP ( 'NONE', ( #19452, #5309, #11785, #6845 ) ) ;
#2855=DIRECTION ( 'NONE',  ( -0.7313537016191773432, 0.6819983600624913711, 1.628001950178159721E-16 ) ) ;
#2889=CARTESIAN_POINT ( 'NONE',  ( 77.42435809754135789, -10.99999999999981526, 6.500000000000123457 ) ) ;
#2891=DIRECTION ( 'NONE',  ( 0.6819983600625060260, 0.7313537016191635765, 6.106365041599011361E-16 ) ) ;
#2895=DIRECTION ( 'NONE',  ( -1.000000000000000000, 1.847414967615758933E-47, -3.885780586188017323E-16 ) ) ;
#2899=VECTOR ( 'NONE', #6721, 1000.000000000000000 ) ;
#2907=VERTEX_POINT ( 'NONE', #21373 ) ;
#2910=ORIENTED_EDGE ( 'NONE', *, *, #4920, .F. ) ;
#2921=LINE ( 'NONE', #1166, #19297 ) ;
#2922=DIRECTION ( 'NONE',  ( -0.7313537016191765661, -0.6819983600624919262, 1.280489736994879814E-15 ) ) ;
#2925=LINE ( 'NONE', #17141, #19348 ) ;
#2928=DIRECTION ( 'NONE',  ( -0.7313537016191730133, 0.6819983600624959230, -5.924440990721418971E-17 ) ) ;
#2934=DIRECTION ( 'NONE',  ( 1.000000000000000000, 5.598259082250514647E-17, 3.330669073875432643E-16 ) ) ;
#2937=EDGE_CURVE ( 'NONE', #5312, #2822, #19856, .T. ) ;
#2942=AXIS2_PLACEMENT_3D ( 'NONE', #22696, #15613, #17138 ) ;
#2963=DIRECTION ( 'NONE',  ( 0.000000000000000000, 0.000000000000000000, 1.000000000000000000 ) ) ;
#2965=EDGE_CURVE ( 'NONE', #8517, #6969, #8583, .T. ) ;
#2970=VERTEX_POINT ( 'NONE', #5837 ) ;
#2977=TOROIDAL_SURFACE ( 'NONE', #16104, 6.500000000000000888, 0.5000000000000000000 ) ;
#2990=LINE ( 'NONE', #10160, #21709 ) ;
#2992=LINE ( 'NONE', #22172, #11157 ) ;
#2995=PRODUCT_DEFINITION_CONTEXT ( 'detailed design', #2765, 'design' ) ;
#2997=EDGE_LOOP ( 'NONE', ( #23121, #6037, #23053, #17300 ) ) ;
#3012=CARTESIAN_POINT ( 'NONE',  ( 54.42435809754113052, -4.000000000000003553, -6.000000000000012434 ) ) ;
#3019=ORIENTED_EDGE ( 'NONE', *, *, #19333, .F. ) ;
#3033=ORIENTED_EDGE ( 'NONE', *, *, #13323, .F. ) ;
#3043=EDGE_CURVE ( 'NONE', #20178, #6413, #22167, .T. ) ;
#3044=CARTESIAN_POINT ( 'NONE',  ( 124.5000000000017195, -4.500000000000059508, 1.387778780781445676E-14 ) ) ;
#3046=DIRECTION ( 'NONE',  ( 1.000000000000000000, 5.598259082250514647E-17, 3.330669073875432643E-16 ) ) ;
#3053=EDGE_CURVE ( 'NONE', #18271, #22610, #763, .T. ) ;
#3076=ADVANCED_FACE ( 'NONE', ( #8160 ), #13459, .T. ) ;
#3100=CIRCLE ( 'NONE', #13970, 7.000000000000075495 ) ;
#3103=CARTESIAN_POINT ( 'NONE',  ( 80.49335071782266482, -7.708908342713566064, -6.500000000000047073 ) ) ;
#3107=CARTESIAN_POINT ( 'NONE',  ( 54.42435809754108078, -4.000000000000003553, 6.500000000000081712 ) ) ;
#3108=FACE_OUTER_BOUND ( 'NONE', #1126, .T. ) ;
#3113=ORIENTED_EDGE ( 'NONE', *, *, #20891, .T. ) ;
#3115=ORIENTED_EDGE ( 'NONE', *, *, #20628, .T. ) ;
#3143=CIRCLE ( 'NONE', #16633, 0.4999999999999990563 ) ;
#3159=AXIS2_PLACEMENT_3D ( 'NONE', #1724, #14314, #8791 ) ;
#3161=DIRECTION ( 'NONE',  ( 3.885780586188016830E-16, 4.437342591868156373E-31, -1.000000000000000000 ) ) ;
#3172=AXIS2_PLACEMENT_3D ( 'NONE', #7552, #18480, #11190 ) ;
#3176=AXIS2_PLACEMENT_3D ( 'NONE', #18080, #11005, #9371 ) ;
#3184=ORIENTED_EDGE ( 'NONE', *, *, #6586, .F. ) ;
#3185=CARTESIAN_POINT ( 'NONE',  ( 2.498001805406602216E-13, 0.000000000000000000, 6.500000000000103029 ) ) ;
#3187=CIRCLE ( 'NONE', #3172, 2.550000000000012701 ) ;
#3192=CARTESIAN_POINT ( 'NONE',  ( 6.500000000000227374, 2.500000000000168754, 4.163336342344337027E-14 ) ) ;
#3196=DIRECTION ( 'NONE',  ( 3.885780586188016830E-16, 4.437342591868156373E-31, -1.000000000000000000 ) ) ;
#3201=DIRECTION ( 'NONE',  ( -4.336808689941983223E-16, 0.000000000000000000, 1.000000000000000000 ) ) ;
#3205=ADVANCED_FACE ( 'NONE', ( #17888 ), #18235, .T. ) ;
#3208=ORIENTED_EDGE ( 'NONE', *, *, #13713, .T. ) ;
#3210=ORIENTED_EDGE ( 'NONE', *, *, #1173, .F. ) ;
#3223=CARTESIAN_POINT ( 'NONE',  ( 88.75737332930596324, -13.02760560296348302, -6.499999999999964473 ) ) ;
#3225=AXIS2_PLACEMENT_3D ( 'NONE', #3185, #10342, #5643 ) ;
#3232=CARTESIAN_POINT ( 'NONE',  ( 108.2426266706970637, -13.02760560296348302, 6.500000000000019540 ) ) ;
#3238=ORIENTED_EDGE ( 'NONE', *, *, #16415, .T. ) ;
#3241=ORIENTED_EDGE ( 'NONE', *, *, #21339, .T. ) ;
#3249=AXIS2_PLACEMENT_3D ( 'NONE', #15160, #15387, #22575 ) ;
#3263=FACE_OUTER_BOUND ( 'NONE', #12746, .T. ) ;
#3270=VERTEX_POINT ( 'NONE', #18348 ) ;
#3271=DIRECTION ( 'NONE',  ( 3.885780586188016830E-16, 4.437342591868156373E-31, -1.000000000000000000 ) ) ;
#3272=CARTESIAN_POINT ( 'NONE',  ( 77.42435809754134368, -10.99999999999981526, -6.000000000000047073 ) ) ;
#3286=CARTESIAN_POINT ( 'NONE',  ( 124.5000000000019469, -13.52760560296373171, -2.550000000000019806 ) ) ;
#3287=VECTOR ( 'NONE', #13225, 1000.000000000000000 ) ;
#3288=CARTESIAN_POINT ( 'NONE',  ( 66.26395429947837101, -4.000000000000003553, -5.999999999999956479 ) ) ;
#3291=ORIENTED_EDGE ( 'NONE', *, *, #10387, .F. ) ;
#3298=ORIENTED_EDGE ( 'NONE', *, *, #6520, .T. ) ;
#3300=LINE ( 'NONE', #23184, #14482 ) ;
#3315=CIRCLE ( 'NONE', #2171, 0.5000000000000038858 ) ;
#3321=VERTEX_POINT ( 'NONE', #11278 ) ;
#3327=DIRECTION ( 'NONE',  ( 3.885780586188016830E-16, 4.437342591868156373E-31, -1.000000000000000000 ) ) ;
#3332=VECTOR ( 'NONE', #9653, 1000.000000000000000 ) ;
#3335=DIRECTION ( 'NONE',  ( -3.885780586188016830E-16, -4.437342591868156373E-31, 1.000000000000000000 ) ) ;
#3338=EDGE_CURVE ( 'NONE', #18645, #15739, #6230, .T. ) ;
#3363=DIRECTION ( 'NONE',  ( 1.000000000000000000, 5.598259082250514647E-17, 3.330669073875432643E-16 ) ) ;
#3371=DIRECTION ( 'NONE',  ( 1.000000000000000000, 2.699383410053119644E-30, 3.330669073875432643E-16 ) ) ;
#3374=LINE ( 'NONE', #11937, #18273 ) ;
#3380=ORIENTED_EDGE ( 'NONE', *, *, #10802, .T. ) ;
#3389=FACE_OUTER_BOUND ( 'NONE', #19082, .T. ) ;
#3404=DIRECTION ( 'NONE',  ( 1.000000000000000000, -7.477632011778292156E-48, 3.885780586188017323E-16 ) ) ;
#3441=DIRECTION ( 'NONE',  ( 3.241725282392603095E-30, 1.000000000000000000, -2.218671295934100958E-31 ) ) ;
#3457=EDGE_LOOP ( 'NONE', ( #6063, #11657, #9748, #12715 ) ) ;
#3460=ORIENTED_EDGE ( 'NONE', *, *, #21410, .F. ) ;
#3464=ORIENTED_EDGE ( 'NONE', *, *, #18747, .F. ) ;
#3473=FACE_OUTER_BOUND ( 'NONE', #2172, .T. ) ;
#3487=AXIS2_PLACEMENT_3D ( 'NONE', #1947, #5618, #2188 ) ;
#3496=FACE_OUTER_BOUND ( 'NONE', #2492, .T. ) ;
#3505=DIRECTION ( 'NONE',  ( 1.000000000000000000, 2.699383410053117892E-30, 3.885780586188017323E-16 ) ) ;
#3506=ADVANCED_FACE ( 'NONE', ( #10104 ), #17377, .T. ) ;
#3508=PLANE ( 'NONE',  #18983 ) ;
#3514=CARTESIAN_POINT ( 'NONE',  ( 63.53596085922837489, -2.925414806476733798, -6.499999999999957367 ) ) ;
#3530=DIRECTION ( 'NONE',  ( -1.000000000000000000, -2.699383410053119644E-30, -3.330669073875432643E-16 ) ) ;
#3549=ORIENTED_EDGE ( 'NONE', *, *, #4802, .F. ) ;
#3552=EDGE_LOOP ( 'NONE', ( #11060, #2796, #4284, #4278 ) ) ;
#3587=AXIS2_PLACEMENT_3D ( 'NONE', #3044, #8332, #6580 ) ;
#3591=DIRECTION ( 'NONE',  ( 3.885780586188016830E-16, 4.437342591868156373E-31, -1.000000000000000000 ) ) ;
#3603=ORIENTED_EDGE ( 'NONE', *, *, #6089, .F. ) ;
#3605=ADVANCED_FACE ( 'NONE', ( #7165 ), #14093, .T. ) ;
#3616=DIRECTION ( 'NONE',  ( 3.885780586188016830E-16, 4.437342591868156373E-31, -1.000000000000000000 ) ) ;
#3619=DIRECTION ( 'NONE',  ( 3.885780586188016830E-16, 4.437342591868156373E-31, -1.000000000000000000 ) ) ;
#3631=FACE_OUTER_BOUND ( 'NONE', #6559, .T. ) ;
#3632=FACE_BOUND ( 'NONE', #11089, .T. ) ;
#3634=VERTEX_POINT ( 'NONE', #12666 ) ;
#3642=AXIS2_PLACEMENT_3D ( 'NONE', #12147, #21464, #23116 ) ;
#3654=CARTESIAN_POINT ( 'NONE',  ( 112.6756160111033722, -11.28140466348817661, 6.500000000000088818 ) ) ;
#3671=FACE_BOUND ( 'NONE', #20070, .T. ) ;
#3672=AXIS2_PLACEMENT_3D ( 'NONE', #6748, #1567, #10507 ) ;
#3679=CARTESIAN_POINT ( 'NONE',  ( 86.31951208941929110, -13.14189171599983119, 6.000000000000109246 ) ) ;
#3682=CARTESIAN_POINT ( 'NONE',  ( 111.0000000000017764, -13.52760560296359316, 6.500000000000068390 ) ) ;
#3703=CARTESIAN_POINT ( 'NONE',  ( 110.9706201109471522, -13.02760560296367665, 6.000000000000088818 ) ) ;
#3710=AXIS2_PLACEMENT_3D ( 'NONE', #19387, #21284, #3404 ) ;
#3712=FACE_OUTER_BOUND ( 'NONE', #1331, .T. ) ;
#3721=CARTESIAN_POINT ( 'NONE',  ( 124.5000000000017195, -4.000000000000058620, 2.550000000000026468 ) ) ;
#3730=CARTESIAN_POINT ( 'NONE',  ( 108.2426266706970637, -13.52760560296348302, 6.500000000000019540 ) ) ;
#3749=DIRECTION ( 'NONE',  ( -1.000000000000000000, 0.000000000000000000, -3.717264591378832268E-16 ) ) ;
#3767=ORIENTED_EDGE ( 'NONE', *, *, #12537, .F. ) ;
#3785=DIRECTION ( 'NONE',  ( 0.000000000000000000, 0.000000000000000000, 1.000000000000000000 ) ) ;
#3804=ORIENTED_EDGE ( 'NONE', *, *, #20917, .F. ) ;
#3814=CARTESIAN_POINT ( 'NONE',  ( 88.75737332930586376, -11.02760560296348125, 6.000000000000165201 ) ) ;
#3823=AXIS2_PLACEMENT_3D ( 'NONE', #7895, #18714, #11645 ) ;
#3828=DIRECTION ( 'NONE',  ( -3.885780586188016830E-16, -4.437342591868156373E-31, 1.000000000000000000 ) ) ;
#3842=AXIS2_PLACEMENT_3D ( 'NONE', #4437, #2804, #934 ) ;
#3844=CIRCLE ( 'NONE', #22257, 7.000000000000075495 ) ;
#3847=ORIENTED_EDGE ( 'NONE', *, *, #3053, .F. ) ;
#3851=CARTESIAN_POINT ( 'NONE',  ( 110.6590008199704869, -13.16192875215410574, -6.000000000000047073 ) ) ;
#3853=CIRCLE ( 'NONE', #5001, 0.5000000000000038858 ) ;
#3855=AXIS2_PLACEMENT_3D ( 'NONE', #6308, #7834, #6542 ) ;
#3856=VECTOR ( 'NONE', #16275, 1000.000000000000000 ) ;
#3860=CARTESIAN_POINT ( 'NONE',  ( 57.15235153779110533, -1.074585193523325266, 6.500000000000117240 ) ) ;
#3862=FACE_OUTER_BOUND ( 'NONE', #7428, .T. ) ;
#3872=VECTOR ( 'NONE', #2928, 1000.000000000000114 ) ;
#3875=CIRCLE ( 'NONE', #22689, 0.5000000000000038858 ) ;
#3880=ORIENTED_EDGE ( 'NONE', *, *, #16542, .F. ) ;
#3884=ORIENTED_EDGE ( 'NONE', *, *, #16127, .T. ) ;
#3885=DIRECTION ( 'NONE',  ( -3.885780586188016830E-16, -4.437342591868156373E-31, 1.000000000000000000 ) ) ;
#3887=EDGE_CURVE ( 'NONE', #10913, #15916, #10301, .T. ) ;
#3889=VECTOR ( 'NONE', #16964, 1000.000000000000000 ) ;
#3922=EDGE_CURVE ( 'NONE', #16601, #15739, #8891, .T. ) ;
#3948=ORIENTED_EDGE ( 'NONE', *, *, #15817, .F. ) ;
#3949=ORIENTED_EDGE ( 'NONE', *, *, #9809, .T. ) ;
#3957=LINE ( 'NONE', #21847, #11492 ) ;
#3960=AXIS2_PLACEMENT_3D ( 'NONE', #17877, #10574, #14232 ) ;
#3965=VECTOR ( 'NONE', #15778, 1000.000000000000000 ) ;
#3977=LINE ( 'NONE', #9403, #12829 ) ;
#3980=CARTESIAN_POINT ( 'NONE',  ( 108.2426266706970353, -11.02760560296359138, -6.000000000000019540 ) ) ;
#3987=FACE_OUTER_BOUND ( 'NONE', #12599, .T. ) ;
#3995=CIRCLE ( 'NONE', #4359, 0.5000000000000038858 ) ;
#3997=EDGE_LOOP ( 'NONE', ( #8633, #17846, #6661, #1968 ) ) ;
#4003=ORIENTED_EDGE ( 'NONE', *, *, #11324, .F. ) ;
#4022=AXIS2_PLACEMENT_3D ( 'NONE', #4910, #11626, #19158 ) ;
#4028=ORIENTED_EDGE ( 'NONE', *, *, #13447, .T. ) ;
#4030=AXIS2_PLACEMENT_3D ( 'NONE', #2106, #1871, #9055 ) ;
#4061=VECTOR ( 'NONE', #19050, 1000.000000000000000 ) ;
#4062=VERTEX_POINT ( 'NONE', #12763 ) ;
#4097=DIRECTION ( 'NONE',  ( 0.000000000000000000, 0.000000000000000000, 1.000000000000000000 ) ) ;
#4104=DIRECTION ( 'NONE',  ( -3.241725282392603095E-30, -1.000000000000000000, 2.218671295934100958E-31 ) ) ;
#4128=CARTESIAN_POINT ( 'NONE',  ( 55.36587326203800075, 4.009651402420072230, -6.499999999999977796 ) ) ;
#4143=CARTESIAN_POINT ( 'NONE',  ( 113.0166151911345906, -11.64708151429785765, 6.000000000000067502 ) ) ;
#4154=CARTESIAN_POINT ( 'NONE',  ( 119.5756419024615838, -7.000000000000062172, -6.000000000000019540 ) ) ;
#4164=VERTEX_POINT ( 'NONE', #21714 ) ;
#4169=VERTEX_POINT ( 'NONE', #5603 ) ;
#4175=EDGE_CURVE ( 'NONE', #12275, #9470, #5943, .T. ) ;
#4202=CARTESIAN_POINT ( 'NONE',  ( 73.50000000000116529, -13.52760560296348302, 2.550000000000047340 ) ) ;
#4204=AXIS2_PLACEMENT_3D ( 'NONE', #19254, #10319, #8794 ) ;
#4235=DIRECTION ( 'NONE',  ( -0.7313537016191730133, 0.6819983600624958120, -5.924440990721418971E-17 ) ) ;
#4243=CARTESIAN_POINT ( 'NONE',  ( 119.5756419024615838, -6.500000000000061284, -6.499999999999992006 ) ) ;
#4247=ORIENTED_EDGE ( 'NONE', *, *, #8981, .T. ) ;
#4251=EDGE_LOOP ( 'NONE', ( #18817, #5197, #13985, #2641 ) ) ;
#4257=CIRCLE ( 'NONE', #17817, 2.550000000000012701 ) ;
#4261=DIRECTION ( 'NONE',  ( -1.000000000000000000, -2.699383410053119644E-30, -3.330669073875432643E-16 ) ) ;
#4263=PLANE ( 'NONE',  #10034 ) ;
#4278=ORIENTED_EDGE ( 'NONE', *, *, #7805, .T. ) ;
#4280=ORIENTED_EDGE ( 'NONE', *, *, #6444, .T. ) ;
#4284=ORIENTED_EDGE ( 'NONE', *, *, #9354, .F. ) ;
#4287=CARTESIAN_POINT ( 'NONE',  ( 111.3116192909783990, -9.818697260249948044, 6.000000000000074607 ) ) ;
#4292=CARTESIAN_POINT ( 'NONE',  ( 82.19834661797897013, -6.499999999999811706, 6.000000000000109246 ) ) ;
#4300=CARTESIAN_POINT ( 'NONE',  ( 66.26395429947837101, -4.500000000000003553, -5.999999999999956479 ) ) ;
#4310=VERTEX_POINT ( 'NONE', #8047 ) ;
#4313=CARTESIAN_POINT ( 'NONE',  ( 88.75737332930597745, -13.52760560296348302, -6.000000000000039968 ) ) ;
#4319=DIRECTION ( 'NONE',  ( -1.000000000000000000, 1.598721155460238356E-14, -3.717264591378832268E-16 ) ) ;
#4321=EDGE_CURVE ( 'NONE', #4634, #7123, #7928, .T. ) ;
#4325=CARTESIAN_POINT ( 'NONE',  ( 124.5000000000017195, -4.500000000000059508, 1.387778780781445676E-14 ) ) ;
#4333=ORIENTED_EDGE ( 'NONE', *, *, #20748, .T. ) ;
#4337=CARTESIAN_POINT ( 'NONE',  ( 88.75737332930587797, -10.52760560296347947, 6.500000000000075495 ) ) ;
#4352=SURFACE_STYLE_FILL_AREA ( #11195 ) ;
#4357=DIRECTION ( 'NONE',  ( -1.000000000000000000, -5.598259082250514647E-17, -3.330669073875432643E-16 ) ) ;
#4359=AXIS2_PLACEMENT_3D ( 'NONE', #15235, #19128, #6435 ) ;
#4368=ORIENTED_EDGE ( 'NONE', *, *, #2209, .T. ) ;
#4387=CARTESIAN_POINT ( 'NONE',  ( 108.2426266706970637, -11.02760560296348125, 6.500000000000019540 ) ) ;
#4388=CARTESIAN_POINT ( 'NONE',  ( 66.26395429947838522, 0.000000000000000000, 6.500000000000144773 ) ) ;
#4395=ORIENTED_EDGE ( 'NONE', *, *, #2261, .T. ) ;
#4404=VECTOR ( 'NONE', #18043, 1000.000000000000000 ) ;
#4406=ORIENTED_EDGE ( 'NONE', *, *, #1271, .F. ) ;
#4416=CARTESIAN_POINT ( 'NONE',  ( 119.5756419024615553, -4.500000000000003553, 6.000000000000136779 ) ) ;
#4426=CYLINDRICAL_SURFACE ( 'NONE', #10424, 0.5000000000000025535 ) ;
#4431=ORIENTED_EDGE ( 'NONE', *, *, #8397, .F. ) ;
#4437=CARTESIAN_POINT ( 'NONE',  ( 66.26395429947837101, -6.500000000000005329, -5.999999999999956479 ) ) ;
#4443=AXIS2_PLACEMENT_3D ( 'NONE', #468, #2458, #15037 ) ;
#4446=CARTESIAN_POINT ( 'NONE',  ( 66.26395429947837101, -6.500000000000005329, 6.500000000000110134 ) ) ;
#4447=FACE_OUTER_BOUND ( 'NONE', #13813, .T. ) ;
#4458=EDGE_CURVE ( 'NONE', #14358, #7123, #16768, .T. ) ;
#4459=ORIENTED_EDGE ( 'NONE', *, *, #14111, .T. ) ;
#4462=ORIENTED_EDGE ( 'NONE', *, *, #8114, .F. ) ;
#4463=ORIENTED_EDGE ( 'NONE', *, *, #18024, .F. ) ;
#4469=LINE ( 'NONE', #21898, #3332 ) ;
#4474=CIRCLE ( 'NONE', #17627, 0.5000000000000031086 ) ;
#4491=EDGE_CURVE ( 'NONE', #4310, #10913, #11145, .T. ) ;
#4493=ORIENTED_EDGE ( 'NONE', *, *, #22019, .F. ) ;
#4507=EDGE_CURVE ( 'NONE', #13843, #11516, #22812, .T. ) ;
#4508=DIRECTION ( 'NONE',  ( -1.000000000000000000, -2.699383410053119644E-30, -3.330669073875432643E-16 ) ) ;
#4515=DIRECTION ( 'NONE',  ( 3.885780586188016830E-16, 4.437342591868156373E-31, -1.000000000000000000 ) ) ;
#4516=EDGE_CURVE ( 'NONE', #17475, #3321, #20266, .T. ) ;
#4545=CARTESIAN_POINT ( 'NONE',  ( 77.42435809754145737, -4.499999999999809930, -6.499999999999984901 ) ) ;
#4553=DIRECTION ( 'NONE',  ( -3.885780586188016830E-16, -4.437342591868156373E-31, 1.000000000000000000 ) ) ;
#4556=DIRECTION ( 'NONE',  ( 0.7313537016191746787, 0.6819983600624940356, 1.072890437865584409E-16 ) ) ;
#4564=LINE ( 'NONE', #6234, #6291 ) ;
#4573=ORIENTED_EDGE ( 'NONE', *, *, #4516, .F. ) ;
#4581=CARTESIAN_POINT ( 'NONE',  ( 116.5066492821803052, -7.708908342713815642, -6.500000000000005329 ) ) ;
#4587=FACE_OUTER_BOUND ( 'NONE', #2997, .T. ) ;
#4594=DIRECTION ( 'NONE',  ( 1.000000000000000000, 2.699383410053119644E-30, 3.330669073875432643E-16 ) ) ;
#4601=ORIENTED_EDGE ( 'NONE', *, *, #18024, .T. ) ;
#4606=VERTEX_POINT ( 'NONE', #11298 ) ;
#4608=FACE_OUTER_BOUND ( 'NONE', #22785, .T. ) ;
#4609=CYLINDRICAL_SURFACE ( 'NONE', #11062, 0.5000000000000038858 ) ;
#4613=AXIS2_PLACEMENT_3D ( 'NONE', #8528, #7010, #7134 ) ;
#4621=DIRECTION ( 'NONE',  ( -1.000000000000000000, -2.699383410053119644E-30, -3.330669073875432643E-16 ) ) ;
#4629=ORIENTED_EDGE ( 'NONE', *, *, #23195, .T. ) ;
#4634=VERTEX_POINT ( 'NONE', #5900 ) ;
#4654=CARTESIAN_POINT ( 'NONE',  ( 66.26395429947839943, 0.000000000000000000, 6.000000000000178524 ) ) ;
#4663=CARTESIAN_POINT ( 'NONE',  ( 77.42435809754134368, -10.99999999999981526, -6.000000000000047073 ) ) ;
#4680=EDGE_LOOP ( 'NONE', ( #7094, #1812, #4864, #11174 ) ) ;
#4689=ADVANCED_FACE ( 'NONE', ( #2705 ), #5156, .T. ) ;
#4705=ORIENTED_EDGE ( 'NONE', *, *, #9638, .T. ) ;
#4716=CARTESIAN_POINT ( 'NONE',  ( 84.32438398889955522, -11.28140466348809312, 6.000000000000095923 ) ) ;
#4732=DIRECTION ( 'NONE',  ( 0.000000000000000000, 0.000000000000000000, 1.000000000000000000 ) ) ;
#4733=DIRECTION ( 'NONE',  ( 3.032184104443271834E-30, 1.000000000000000000, 4.437342591868167759E-31 ) ) ;
#4734=AXIS2_PLACEMENT_3D ( 'NONE', #10786, #13023, #3505 ) ;
#4750=EDGE_LOOP ( 'NONE', ( #23267, #3208, #14511, #14160 ) ) ;
#4762=CARTESIAN_POINT ( 'NONE',  ( 57.15235153779114796, -1.074585193523325266, -6.499999999999977796 ) ) ;
#4766=CARTESIAN_POINT ( 'NONE',  ( 108.2426266706970353, -6.527605602963587828, 6.500000000000199840 ) ) ;
#4773=CIRCLE ( 'NONE', #20940, 4.500000000000045297 ) ;
#4776=COLOUR_RGB ( '', 0.09019608, 0.27058824, 0.51372549) ;
#4780=TOROIDAL_SURFACE ( 'NONE', #17942, 4.500000000000000888, 0.5000000000000000000 ) ;
#4791=DIRECTION ( 'NONE',  ( 3.885780586188016830E-16, 4.437342591868156373E-31, -1.000000000000000000 ) ) ;
#4793=DIRECTION ( 'NONE',  ( -1.000000000000000000, 0.000000000000000000, -2.668805347656595124E-16 ) ) ;
#4802=EDGE_CURVE ( 'NONE', #9470, #7130, #12783, .T. ) ;
#4815=ORIENTED_EDGE ( 'NONE', *, *, #13276, .F. ) ;
#4838=ORIENTED_EDGE ( 'NONE', *, *, #5054, .T. ) ;
#4842=ORIENTED_EDGE ( 'NONE', *, *, #8094, .F. ) ;
#4844=DIRECTION ( 'NONE',  ( -1.000000000000000000, 0.000000000000000000, -3.717264591378832268E-16 ) ) ;
#4858=FACE_OUTER_BOUND ( 'NONE', #2665, .T. ) ;
#4864=ORIENTED_EDGE ( 'NONE', *, *, #12932, .F. ) ;
#4874=EDGE_CURVE ( 'NONE', #5583, #18644, #3957, .T. ) ;
#4878=PLANE ( 'NONE',  #5712 ) ;
#4897=VECTOR ( 'NONE', #11641, 1000.000000000000000 ) ;
#4899=CARTESIAN_POINT ( 'NONE',  ( 58.04599508018838350, 2.194061104857397915, -5.999999999999991118 ) ) ;
#4903=PLANE ( 'NONE',  #16070 ) ;
#4910=CARTESIAN_POINT ( 'NONE',  ( 73.50000000000115108, -6.999999999999811706, -6.938893903907228378E-15 ) ) ;
#4912=ADVANCED_FACE ( 'NONE', ( #5858 ), #15627, .T. ) ;
#4920=EDGE_CURVE ( 'NONE', #8376, #22529, #17505, .T. ) ;
#4927=FACE_OUTER_BOUND ( 'NONE', #20163, .T. ) ;
#4929=VERTEX_POINT ( 'NONE', #2659 ) ;
#4933=DIRECTION ( 'NONE',  ( 1.000000000000000000, 2.699383410053119644E-30, 3.330669073875432643E-16 ) ) ;
#4940=CARTESIAN_POINT ( 'NONE',  ( 61.48996577904082272, -5.119475911334187224, -5.999999999999928946 ) ) ;
#4943=CARTESIAN_POINT ( 'NONE',  ( 0.000000000000000000, 0.000000000000000000, 0.000000000000000000 ) ) ;
#4956=DIRECTION ( 'NONE',  ( 0.000000000000000000, 0.000000000000000000, 1.000000000000000000 ) ) ;
#4961=CARTESIAN_POINT ( 'NONE',  ( 54.42435809754109499, 0.000000000000000000, 6.500000000000144773 ) ) ;
#4978=AXIS2_PLACEMENT_3D ( 'NONE', #3679, #4235, #7777 ) ;
#4993=PLANE ( 'NONE',  #1860 ) ;
#5001=AXIS2_PLACEMENT_3D ( 'NONE', #8248, #13539, #10011 ) ;
#5005=AXIS2_PLACEMENT_3D ( 'NONE', #7440, #5681, #20021 ) ;
#5013=ADVANCED_FACE ( 'NONE', ( #6893 ), #14067, .F. ) ;
#5015=EDGE_CURVE ( 'NONE', #11319, #17475, #3374, .T. ) ;
#5018=FACE_OUTER_BOUND ( 'NONE', #12799, .T. ) ;
#5023=VECTOR ( 'NONE', #20822, 1000.000000000000000 ) ;
#5027=AXIS2_PLACEMENT_3D ( 'NONE', #1075, #13651, #19057 ) ;
#5037=LINE ( 'NONE', #3286, #7735 ) ;
#5040=CIRCLE ( 'NONE', #16319, 6.500000000000075495 ) ;
#5054=EDGE_CURVE ( 'NONE', #20178, #6969, #17771, .T. ) ;
#5056=CARTESIAN_POINT ( 'NONE',  ( 73.50000000000116529, -6.999999999999811706, 2.549999999999985612 ) ) ;
#5058=CARTESIAN_POINT ( 'NONE',  ( 61.83096495907212642, -4.753799060524616316, -6.500000000000012434 ) ) ;
#5059=CIRCLE ( 'NONE', #13711, 6.500000000000075495 ) ;
#5079=EDGE_CURVE ( 'NONE', #11319, #16591, #12502, .T. ) ;
#5085=EDGE_CURVE ( 'NONE', #15653, #5583, #16624, .T. ) ;
#5088=DIRECTION ( 'NONE',  ( 0.000000000000000000, 0.000000000000000000, 1.000000000000000000 ) ) ;
#5090=CARTESIAN_POINT ( 'NONE',  ( 112.6756160111034575, -11.28140466348828674, -6.500000000000040856 ) ) ;
#5100=DIRECTION ( 'NONE',  ( 3.885780586188016830E-16, 4.437342591868156373E-31, -1.000000000000000000 ) ) ;
#5109=ORIENTED_EDGE ( 'NONE', *, *, #3922, .F. ) ;
#5111=FACE_OUTER_BOUND ( 'NONE', #8816, .T. ) ;
#5116=CARTESIAN_POINT ( 'NONE',  ( 57.15235153779116217, -1.074585193523325266, -5.999999999999894307 ) ) ;
#5118=DIRECTION ( 'NONE',  ( -1.000000000000000000, 1.771896121890576795E-14, -3.717264591378832268E-16 ) ) ;
#5123=DIRECTION ( 'NONE',  ( 1.000000000000000000, 2.699383410053119644E-30, 3.330669073875432643E-16 ) ) ;
#5125=CARTESIAN_POINT ( 'NONE',  ( 124.5000000000018332, -4.500000000000059508, -5.999999999999943157 ) ) ;
#5126=FACE_OUTER_BOUND ( 'NONE', #14994, .T. ) ;
#5131=DIRECTION ( 'NONE',  ( -1.000000000000000000, -2.699383410053119644E-30, -3.330669073875432643E-16 ) ) ;
#5137=AXIS2_PLACEMENT_3D ( 'NONE', #23228, #21576, #17806 ) ;
#5139=EDGE_CURVE ( 'NONE', #13451, #18021, #11104, .T. ) ;
#5140=ORIENTED_EDGE ( 'NONE', *, *, #14573, .T. ) ;
#5141=DIRECTION ( 'NONE',  ( -0.7313537016191735685, 0.6819983600624951459, -3.923113172947598083E-16 ) ) ;
#5154=AXIS2_PLACEMENT_3D ( 'NONE', #6836, #8485, #8135 ) ;
#5155=DIRECTION ( 'NONE',  ( -1.000000000000000000, -2.699383410053119644E-30, -3.330669073875432643E-16 ) ) ;
#5156=TOROIDAL_SURFACE ( 'NONE', #18304, 6.500000000000000888, 0.5000000000000000000 ) ;
#5161=CARTESIAN_POINT ( 'NONE',  ( 118.0000000000019043, -7.000000000000006217, 6.500000000000103029 ) ) ;
#5163=ORIENTED_EDGE ( 'NONE', *, *, #11403, .T. ) ;
#5167=ORIENTED_EDGE ( 'NONE', *, *, #14686, .T. ) ;
#5175=AXIS2_PLACEMENT_3D ( 'NONE', #23231, #21347, #20030 ) ;
#5179=FACE_OUTER_BOUND ( 'NONE', #22067, .T. ) ;
#5182=EDGE_CURVE ( 'NONE', #18271, #18021, #21529, .T. ) ;
#5192=( LENGTH_UNIT ( ) NAMED_UNIT ( * ) SI_UNIT ( .MILLI., .METRE. ) );
#5197=ORIENTED_EDGE ( 'NONE', *, *, #12242, .T. ) ;
#5199=ORIENTED_EDGE ( 'NONE', *, *, #20779, .T. ) ;
#5200=EDGE_LOOP ( 'NONE', ( #8149, #1827, #20970, #2845 ) ) ;
#5203=STYLED_ITEM ( 'NONE', ( #9734 ), #22653 ) ;
#5204=PLANE ( 'NONE',  #22363 ) ;
#5206=CARTESIAN_POINT ( 'NONE',  ( 86.00000000000129319, -10.52760560296347947, 6.500000000000110134 ) ) ;
#5212=PLANE ( 'NONE',  #18524 ) ;
#5217=CARTESIAN_POINT ( 'NONE',  ( 66.26395429947838522, 0.000000000000000000, -6.499999999999859668 ) ) ;
#5224=FACE_OUTER_BOUND ( 'NONE', #12004, .T. ) ;
#5256=VERTEX_POINT ( 'NONE', #11450 ) ;
#5265=EDGE_LOOP ( 'NONE', ( #20009, #12578, #19806, #17128 ) ) ;
#5290=CARTESIAN_POINT ( 'NONE',  ( 59.19834661797866460, 1.119475911334100182, 6.500000000000130562 ) ) ;
#5296=DIRECTION ( 'NONE',  ( -5.598259082250079541E-17, 1.000000000000000000, -6.162975822039171151E-32 ) ) ;
#5306=DIRECTION ( 'NONE',  ( 1.000000000000000000, 0.000000000000000000, 0.000000000000000000 ) ) ;
#5309=ORIENTED_EDGE ( 'NONE', *, *, #22914, .T. ) ;
#5312=VERTEX_POINT ( 'NONE', #3103 ) ;
#5316=CIRCLE ( 'NONE', #21486, 6.500000000000067502 ) ;
#5321=CARTESIAN_POINT ( 'NONE',  ( 108.2426266706970637, -6.527605602963671316, -5.999999999999991118 ) ) ;
#5341=EDGE_CURVE ( 'NONE', #22506, #17475, #1950, .T. ) ;
#5342=ORIENTED_EDGE ( 'NONE', *, *, #11839, .F. ) ;
#5349=VERTEX_POINT ( 'NONE', #22630 ) ;
#5352=TOROIDAL_SURFACE ( 'NONE', #8346, 4.500000000000000888, 0.5000000000000000000 ) ;
#5358=AXIS2_PLACEMENT_3D ( 'NONE', #14441, #16183, #21512 ) ;
#5383=ORIENTED_EDGE ( 'NONE', *, *, #20439, .T. ) ;
#5407=AXIS2_PLACEMENT_3D ( 'NONE', #20110, #7526, #5999 ) ;
#5411=CIRCLE ( 'NONE', #1660, 0.5000000000000031086 ) ;
#5414=ORIENTED_EDGE ( 'NONE', *, *, #11782, .T. ) ;
#5422=FACE_OUTER_BOUND ( 'NONE', #22497, .T. ) ;
#5441=ORIENTED_EDGE ( 'NONE', *, *, #5944, .T. ) ;
#5469=EDGE_LOOP ( 'NONE', ( #11756, #4838, #4003, #3949 ) ) ;
#5474=DIRECTION ( 'NONE',  ( 0.000000000000000000, 0.000000000000000000, 1.000000000000000000 ) ) ;
#5478=CYLINDRICAL_SURFACE ( 'NONE', #23055, 0.5000000000000038858 ) ;
#5485=ORIENTED_EDGE ( 'NONE', *, *, #12201, .T. ) ;
#5496=CARTESIAN_POINT ( 'NONE',  ( 88.75737332930592061, -6.527605602963476805, -6.000000000000012434 ) ) ;
#5519=ORIENTED_EDGE ( 'NONE', *, *, #15983, .T. ) ;
#5524=DIRECTION ( 'NONE',  ( -3.241725282392603095E-30, -1.000000000000000000, 2.218671295934100958E-31 ) ) ;
#5530=EDGE_CURVE ( 'NONE', #4164, #2826, #1967, .T. ) ;
#5539=CARTESIAN_POINT ( 'NONE',  ( 54.42435809754109499, 0.000000000000000000, 6.500000000000144773 ) ) ;
#5540=ADVANCED_FACE ( 'NONE', ( #7215 ), #14379, .T. ) ;
#5561=FACE_OUTER_BOUND ( 'NONE', #5851, .T. ) ;
#5569=CARTESIAN_POINT ( 'NONE',  ( 54.42435809754108078, -4.000000000000003553, 6.500000000000081712 ) ) ;
#5583=VERTEX_POINT ( 'NONE', #2369 ) ;
#5595=CARTESIAN_POINT ( 'NONE',  ( 66.26395429947837101, 0.000000000000000000, -5.999999999999908518 ) ) ;
#5603=CARTESIAN_POINT ( 'NONE',  ( 119.5756419024615553, -4.000000000000003553, 6.000000000000136779 ) ) ;
#5606=VERTEX_POINT ( 'NONE', #16704 ) ;
#5614=ORIENTED_EDGE ( 'NONE', *, *, #15451, .F. ) ;
#5618=DIRECTION ( 'NONE',  ( 3.885780586188016830E-16, 4.437342591868156373E-31, -1.000000000000000000 ) ) ;
#5625=DIRECTION ( 'NONE',  ( 0.7313537016191733464, -0.6819983600624954789, 3.733258675956564523E-18 ) ) ;
#5629=CARTESIAN_POINT ( 'NONE',  ( 88.75737332930594903, -13.52760560296348302, 6.000000000000130562 ) ) ;
#5643=DIRECTION ( 'NONE',  ( -3.885780586188016830E-16, -4.437342591868156373E-31, 1.000000000000000000 ) ) ;
#5645=EDGE_CURVE ( 'NONE', #2907, #14077, #16233, .T. ) ;
#5657=CARTESIAN_POINT ( 'NONE',  ( 85.68838070902455684, -9.818697260249752645, 6.500000000000158096 ) ) ;
#5659=CARTESIAN_POINT ( 'NONE',  ( 124.5000000000019469, -7.000000000000062172, 2.550000000000033573 ) ) ;
#5667=ORIENTED_EDGE ( 'NONE', *, *, #5085, .F. ) ;
#5671=PLANE ( 'NONE',  #8418 ) ;
#5681=DIRECTION ( 'NONE',  ( -3.885780586188016830E-16, -4.437342591868156373E-31, 1.000000000000000000 ) ) ;
#5693=ORIENTED_EDGE ( 'NONE', *, *, #519, .F. ) ;
#5712=AXIS2_PLACEMENT_3D ( 'NONE', #9960, #10297, #12047 ) ;
#5714=DIRECTION ( 'NONE',  ( 1.000000000000000000, -1.847414967615758933E-47, 3.885780586188017323E-16 ) ) ;
#5715=DIRECTION ( 'NONE',  ( 1.000000000000000000, 2.699383410053119644E-30, 3.330669073875432643E-16 ) ) ;
#5720=DIRECTION ( 'NONE',  ( 3.885780586188016830E-16, 4.437342591868156373E-31, -1.000000000000000000 ) ) ;
#5727=ORIENTED_EDGE ( 'NONE', *, *, #22746, .T. ) ;
#5752=CARTESIAN_POINT ( 'NONE',  ( 84.32438398889952680, -11.28140466348809312, 6.500000000000137668 ) ) ;
#5766=DIRECTION ( 'NONE',  ( 3.885780586188016830E-16, 4.437342591868156373E-31, -1.000000000000000000 ) ) ;
#5768=DIRECTION ( 'NONE',  ( 3.885780586188016830E-16, 4.437342591868156373E-31, -1.000000000000000000 ) ) ;
#5780=ADVANCED_FACE ( 'NONE', ( #8254 ), #22104, .T. ) ;
#5800=FACE_OUTER_BOUND ( 'NONE', #6910, .T. ) ;
#5801=DIRECTION ( 'NONE',  ( -0.7313537016191745677, -0.6819983600624940356, -1.072890437865584285E-16 ) ) ;
#5814=ADVANCED_FACE ( 'NONE', ( #19651 ), #8836, .T. ) ;
#5827=EDGE_LOOP ( 'NONE', ( #7002, #15717, #1934, #10316 ) ) ;
#5828=ORIENTED_EDGE ( 'NONE', *, *, #10930, .F. ) ;
#5837=CARTESIAN_POINT ( 'NONE',  ( 63.53596085922831804, -2.925414806476678287, 6.000000000000136779 ) ) ;
#5848=ORIENTED_EDGE ( 'NONE', *, *, #5015, .T. ) ;
#5851=EDGE_LOOP ( 'NONE', ( #9186, #13745, #21418, #10932 ) ) ;
#5854=CARTESIAN_POINT ( 'NONE',  ( 6.500000000000005329, 0.5000000000001669775, 3.469446951953614189E-14 ) ) ;
#5858=FACE_OUTER_BOUND ( 'NONE', #9976, .T. ) ;
#5870=CARTESIAN_POINT ( 'NONE',  ( 6.500000000000088818, -13.52760560296348302, 6.500000000000075495 ) ) ;
#5872=DIRECTION ( 'NONE',  ( 3.885780586188016830E-16, 4.437342591868156373E-31, -1.000000000000000000 ) ) ;
#5874=DIRECTION ( 'NONE',  ( 3.885780586188016830E-16, 4.437342591868156373E-31, -1.000000000000000000 ) ) ;
#5900=CARTESIAN_POINT ( 'NONE',  ( 116.8476484622116232, -8.074585193523331483, 6.000000000000136779 ) ) ;
#5901=CYLINDRICAL_SURFACE ( 'NONE', #14059, 6.500000000000067502 ) ;
#5908=STYLED_ITEM ( 'NONE', ( #11302 ), #20836 ) ;
#5919=ORIENTED_EDGE ( 'NONE', *, *, #9519, .F. ) ;
#5927=EDGE_CURVE ( 'NONE', #18277, #18843, #18461, .T. ) ;
#5932=AXIS2_PLACEMENT_3D ( 'NONE', #3980, #2567, #4097 ) ;
#5935=CIRCLE ( 'NONE', #8552, 4.500000000000052403 ) ;
#5943=CIRCLE ( 'NONE', #15674, 0.5000000000000038858 ) ;
#5944=EDGE_CURVE ( 'NONE', #21618, #23117, #16681, .T. ) ;
#5949=FACE_OUTER_BOUND ( 'NONE', #18306, .T. ) ;
#5954=EDGE_CURVE ( 'NONE', #22529, #2822, #16912, .T. ) ;
#5956=ADVANCED_FACE ( 'NONE', ( #21998 ), #16789, .F. ) ;
#5958=VECTOR ( 'NONE', #20473, 1000.000000000000000 ) ;
#5965=( GEOMETRIC_REPRESENTATION_CONTEXT ( 3 ) GLOBAL_UNCERTAINTY_ASSIGNED_CONTEXT ( ( #12621 ) ) GLOBAL_UNIT_ASSIGNED_CONTEXT ( ( #22203, #16107, #11142 ) ) REPRESENTATION_CONTEXT ( 'NONE', 'WORKASPACE' ) );
#5968=CARTESIAN_POINT ( 'NONE',  ( 111.3116192909783848, -9.818697260249948044, -6.000000000000067502 ) ) ;
#5973=LINE ( 'NONE', #11253, #2298 ) ;
#5976=VECTOR ( 'NONE', #3371, 1000.000000000000000 ) ;
#5978=FACE_OUTER_BOUND ( 'NONE', #23119, .T. ) ;
#5998=ADVANCED_FACE ( 'NONE', ( #362 ), #9636, .F. ) ;
#5999=DIRECTION ( 'NONE',  ( -1.000000000000000000, 7.477632011778292156E-48, -3.885780586188017323E-16 ) ) ;
#6018=CYLINDRICAL_SURFACE ( 'NONE', #16538, 0.5000000000000038858 ) ;
#6019=CYLINDRICAL_SURFACE ( 'NONE', #11375, 4.000000000000045297 ) ;
#6037=ORIENTED_EDGE ( 'NONE', *, *, #2484, .F. ) ;
#6044=VERTEX_POINT ( 'NONE', #5657 ) ;
#6045=DIRECTION ( 'NONE',  ( -0.6819983600625073583, 0.7313537016191622442, 1.665472943098395307E-16 ) ) ;
#6046=CARTESIAN_POINT ( 'NONE',  ( 115.1426525620553889, -6.246200939475476943, -5.999999999999928946 ) ) ;
#6048=CARTESIAN_POINT ( 'NONE',  ( 124.5000000000019469, -7.000000000000062172, 2.081668171172168513E-14 ) ) ;
#6060=ADVANCED_FACE ( 'NONE', ( #3987 ), #18351, .T. ) ;
#6063=ORIENTED_EDGE ( 'NONE', *, *, #13859, .T. ) ;
#6084=CARTESIAN_POINT ( 'NONE',  ( 119.5756419024615269, -11.00000000000006573, 6.000000000000081712 ) ) ;
#6089=EDGE_CURVE ( 'NONE', #20880, #746, #8924, .T. ) ;
#6093=EDGE_LOOP ( 'NONE', ( #5140, #22640, #12627, #22992 ) ) ;
#6098=EDGE_LOOP ( 'NONE', ( #14620, #17068, #5848, #6440 ) ) ;
#6110=CIRCLE ( 'NONE', #16225, 0.4999999999999990563 ) ;
#6130=VERTEX_POINT ( 'NONE', #13755 ) ;
#6142=CIRCLE ( 'NONE', #22297, 4.500000000000045297 ) ;
#6147=CARTESIAN_POINT ( 'NONE',  ( 54.42435809754115894, 0.000000000000000000, 6.000000000000136779 ) ) ;
#6161=VECTOR ( 'NONE', #11732, 1000.000000000000000 ) ;
#6178=VECTOR ( 'NONE', #10611, 1000.000000000000114 ) ;
#6182=AXIS2_PLACEMENT_3D ( 'NONE', #5496, #14773, #550 ) ;
#6203=EDGE_CURVE ( 'NONE', #13307, #11319, #4564, .T. ) ;
#6204=DIRECTION ( 'NONE',  ( 0.000000000000000000, 0.000000000000000000, 1.000000000000000000 ) ) ;
#6210=ORIENTED_EDGE ( 'NONE', *, *, #8532, .F. ) ;
#6217=FACE_OUTER_BOUND ( 'NONE', #14333, .T. ) ;
#6230=LINE ( 'NONE', #17028, #13058 ) ;
#6232=EDGE_CURVE ( 'NONE', #21954, #11543, #22933, .T. ) ;
#6234=CARTESIAN_POINT ( 'NONE',  ( 57.49335071782242323, -0.7089083427137543580, -6.499999999999922728 ) ) ;
#6245=LINE ( 'NONE', #18945, #22692 ) ;
#6256=DIRECTION ( 'NONE',  ( -3.885780586188016830E-16, -4.437342591868156373E-31, 1.000000000000000000 ) ) ;
#6257=CARTESIAN_POINT ( 'NONE',  ( 108.2426266706970779, -6.527605602963587828, 6.000000000000109246 ) ) ;
#6265=AXIS2_PLACEMENT_3D ( 'NONE', #8657, #12176, #17594 ) ;
#6275=ORIENTED_EDGE ( 'NONE', *, *, #1912, .F. ) ;
#6276=DIRECTION ( 'NONE',  ( 0.000000000000000000, 0.000000000000000000, 1.000000000000000000 ) ) ;
#6291=VECTOR ( 'NONE', #13402, 1000.000000000000114 ) ;
#6299=ORIENTED_EDGE ( 'NONE', *, *, #8397, .T. ) ;
#6308=CARTESIAN_POINT ( 'NONE',  ( 81.85734743794765222, -6.246200939475254899, -5.999999999999921840 ) ) ;
#6331=ORIENTED_EDGE ( 'NONE', *, *, #17861, .T. ) ;
#6340=CARTESIAN_POINT ( 'NONE',  ( 66.26395429947831417, -6.500000000000005329, 6.000000000000192735 ) ) ;
#6344=CARTESIAN_POINT ( 'NONE',  ( 124.5000000000018758, -13.52760560296373171, -6.500000000000081712 ) ) ;
#6358=ORIENTED_EDGE ( 'NONE', *, *, #17948, .F. ) ;
#6362=EDGE_CURVE ( 'NONE', #10913, #7460, #11021, .T. ) ;
#6364=ADVANCED_FACE ( 'NONE', ( #8049 ), #16859, .T. ) ;
#6367=ORIENTED_EDGE ( 'NONE', *, *, #11092, .T. ) ;
#6371=DIRECTION ( 'NONE',  ( -1.000000000000000000, 7.477632011778292156E-48, -3.885780586188017323E-16 ) ) ;
#6389=ADVANCED_FACE ( 'NONE', ( #22285 ), #4780, .T. ) ;
#6391=ORIENTED_EDGE ( 'NONE', *, *, #22914, .F. ) ;
#6392=ADVANCED_FACE ( 'NONE', ( #22519 ), #11453, .F. ) ;
#6393=EDGE_LOOP ( 'NONE', ( #2115, #4280, #2726, #13208 ) ) ;
#6396=DIRECTION ( 'NONE',  ( -0.6819983600624981435, -0.7313537016191709039, 0.000000000000000000 ) ) ;
#6408=DIRECTION ( 'NONE',  ( 1.000000000000000000, 2.699383410053119644E-30, 3.330669073875432643E-16 ) ) ;
#6410=CARTESIAN_POINT ( 'NONE',  ( 66.26395429947838522, 0.000000000000000000, 6.500000000000144773 ) ) ;
#6413=VERTEX_POINT ( 'NONE', #4387 ) ;
#6414=EDGE_LOOP ( 'NONE', ( #6778, #5199, #19809, #861 ) ) ;
#6421=VERTEX_POINT ( 'NONE', #5629 ) ;
#6428=FACE_OUTER_BOUND ( 'NONE', #4251, .T. ) ;
#6434=FACE_OUTER_BOUND ( 'NONE', #6093, .T. ) ;
#6435=DIRECTION ( 'NONE',  ( 0.000000000000000000, 0.000000000000000000, 1.000000000000000000 ) ) ;
#6440=ORIENTED_EDGE ( 'NONE', *, *, #4516, .T. ) ;
#6441=AXIS2_PLACEMENT_3D ( 'NONE', #18454, #22455, #7868 ) ;
#6444=EDGE_CURVE ( 'NONE', #9536, #16601, #19485, .T. ) ;
#6447=DIRECTION ( 'NONE',  ( -0.7313537016191746787, 0.6819983600624942577, -1.502534341919913292E-15 ) ) ;
#6452=DIRECTION ( 'NONE',  ( -1.000000000000000000, -2.699383410053119644E-30, -3.330669073875432643E-16 ) ) ;
#6469=FACE_OUTER_BOUND ( 'NONE', #20742, .T. ) ;
#6474=EDGE_LOOP ( 'NONE', ( #12718, #13781, #12949, #14861 ) ) ;
#6480=AXIS2_PLACEMENT_3D ( 'NONE', #8403, #21230, #13575 ) ;
#6482=DIRECTION ( 'NONE',  ( 3.885780586188016830E-16, 4.437342591868156373E-31, -1.000000000000000000 ) ) ;
#6487=CARTESIAN_POINT ( 'NONE',  ( 80.70499590015747060, -5.171615745951873677, 6.000000000000150990 ) ) ;
#6490=AXIS2_PLACEMENT_3D ( 'NONE', #231, #12802, #2091 ) ;
#6496=VERTEX_POINT ( 'NONE', #12024 ) ;
#6497=VERTEX_POINT ( 'NONE', #6747 ) ;
#6520=EDGE_CURVE ( 'NONE', #17658, #21696, #2990, .T. ) ;
#6525=CIRCLE ( 'NONE', #19671, 6.000000000000063061 ) ;
#6529=ORIENTED_EDGE ( 'NONE', *, *, #19743, .F. ) ;
#6531=AXIS2_PLACEMENT_3D ( 'NONE', #3272, #12187, #18202 ) ;
#6532=VECTOR ( 'NONE', #14801, 1000.000000000000114 ) ;
#6542=DIRECTION ( 'NONE',  ( -0.6819983600624989206, -0.7313537016191700157, 0.000000000000000000 ) ) ;
#6559=EDGE_LOOP ( 'NONE', ( #18846, #16196, #5441, #17131 ) ) ;
#6561=CARTESIAN_POINT ( 'NONE',  ( 54.42435809754118736, 2.499999999999946709, -6.499999999999922728 ) ) ;
#6568=AXIS2_PLACEMENT_3D ( 'NONE', #8039, #15201, #4261 ) ;
#6570=PLANE ( 'NONE',  #17758 ) ;
#6571=CARTESIAN_POINT ( 'NONE',  ( 82.19834661797897013, -5.880524088665628923, -5.999999999999943157 ) ) ;
#6576=LINE ( 'NONE', #15378, #5023 ) ;
#6580=DIRECTION ( 'NONE',  ( 2.242473278838646163E-61, 7.395570986447005381E-32, 1.000000000000000000 ) ) ;
#6586=EDGE_CURVE ( 'NONE', #2826, #4062, #12848, .T. ) ;
#6598=DIRECTION ( 'NONE',  ( 0.6819983600625072473, 0.7313537016191623552, 0.000000000000000000 ) ) ;
#6599=LINE ( 'NONE', #13774, #17385 ) ;
#6602=DIRECTION ( 'NONE',  ( 3.885780586188016830E-16, 4.437342591868156373E-31, -1.000000000000000000 ) ) ;
#6610=AXIS2_PLACEMENT_3D ( 'NONE', #21774, #20116, #22230 ) ;
#6611=EDGE_CURVE ( 'NONE', #18843, #5583, #5935, .T. ) ;
#6613=ORIENTED_EDGE ( 'NONE', *, *, #2062, .F. ) ;
#6631=ORIENTED_EDGE ( 'NONE', *, *, #6663, .F. ) ;
#6634=ORIENTED_EDGE ( 'NONE', *, *, #19473, .T. ) ;
#6642=ORIENTED_EDGE ( 'NONE', *, *, #19743, .T. ) ;
#6644=ADVANCED_FACE ( 'NONE', ( #19801 ), #9087, .F. ) ;
#6651=CARTESIAN_POINT ( 'NONE',  ( 119.5756419024615838, -11.00000000000006573, -6.000000000000116351 ) ) ;
#6653=LINE ( 'NONE', #8306, #10085 ) ;
#6659=ADVANCED_FACE ( 'NONE', ( #10953, #165 ), #19688, .F. ) ;
#6661=ORIENTED_EDGE ( 'NONE', *, *, #19168, .F. ) ;
#6663=EDGE_CURVE ( 'NONE', #9737, #22680, #8984, .T. ) ;
#6666=DIRECTION ( 'NONE',  ( 0.7313537016191735685, -0.6819983600624951459, 3.923113172947598083E-16 ) ) ;
#6678=ADVANCED_FACE ( 'NONE', ( #5224 ), #8183, .T. ) ;
#6689=FACE_OUTER_BOUND ( 'NONE', #10341, .T. ) ;
#6716=MECHANICAL_DESIGN_GEOMETRIC_PRESENTATION_REPRESENTATION('',(#5203),#5965);
#6721=DIRECTION ( 'NONE',  ( 3.032184104443272185E-30, 1.000000000000000000, -7.395570986447005381E-32 ) ) ;
#6747=CARTESIAN_POINT ( 'NONE',  ( 119.5756419024616406, -6.500000000000005329, 6.500000000000151879 ) ) ;
#6748=CARTESIAN_POINT ( 'NONE',  ( 66.26395429947838522, 0.000000000000000000, -6.499999999999859668 ) ) ;
#6753=ORIENTED_EDGE ( 'NONE', *, *, #13810, .T. ) ;
#6767=DIRECTION ( 'NONE',  ( -5.598259082250079541E-17, 1.000000000000000000, -6.162975822039171151E-32 ) ) ;
#6778=ORIENTED_EDGE ( 'NONE', *, *, #21008, .F. ) ;
#6781=DIRECTION ( 'NONE',  ( -1.000000000000000000, -2.699383410053119644E-30, -3.330669073875432643E-16 ) ) ;
#6784=ORIENTED_EDGE ( 'NONE', *, *, #13956, .T. ) ;
#6785=ORIENTED_EDGE ( 'NONE', *, *, #1723, .F. ) ;
#6786=EDGE_CURVE ( 'NONE', #19782, #17658, #2486, .T. ) ;
#6828=VECTOR ( 'NONE', #450, 1000.000000000000000 ) ;
#6836=CARTESIAN_POINT ( 'NONE',  ( 77.42435809754140053, -10.99999999999981526, -6.499999999999999112 ) ) ;
#6845=ORIENTED_EDGE ( 'NONE', *, *, #11582, .T. ) ;
#6849=LINE ( 'NONE', #1553, #12909 ) ;
#6851=CARTESIAN_POINT ( 'NONE',  ( 54.42435809754118736, 2.999999999999947153, -6.499999999999922728 ) ) ;
#6852=DIRECTION ( 'NONE',  ( 0.000000000000000000, 0.000000000000000000, 1.000000000000000000 ) ) ;
#6855=ADVANCED_FACE ( 'NONE', ( #22601 ), #10020, .T. ) ;
#6859=DIRECTION ( 'NONE',  ( 0.000000000000000000, 0.000000000000000000, 1.000000000000000000 ) ) ;
#6871=ORIENTED_EDGE ( 'NONE', *, *, #18748, .F. ) ;
#6893=FACE_OUTER_BOUND ( 'NONE', #22141, .T. ) ;
#6900=CYLINDRICAL_SURFACE ( 'NONE', #6265, 0.4999999999999987232 ) ;
#6902=ORIENTED_EDGE ( 'NONE', *, *, #21008, .T. ) ;
#6907=ORIENTED_EDGE ( 'NONE', *, *, #9301, .F. ) ;
#6910=EDGE_LOOP ( 'NONE', ( #20100, #5109, #246, #3464 ) ) ;
#6917=AXIS2_PLACEMENT_3D ( 'NONE', #11800, #1116, #18988 ) ;
#6919=AXIS2_PLACEMENT_3D ( 'NONE', #6340, #6452, #19040 ) ;
#6924=DIRECTION ( 'NONE',  ( 1.000000000000000000, 4.882007496677533029E-14, 3.717264591378832268E-16 ) ) ;
#6946=CARTESIAN_POINT ( 'NONE',  ( 116.5066492821802768, -7.708908342713760575, 6.500000000000151879 ) ) ;
#6954=CIRCLE ( 'NONE', #16332, 0.4999999999999990563 ) ;
#6967=EDGE_CURVE ( 'NONE', #6496, #18651, #11197, .T. ) ;
#6969=VERTEX_POINT ( 'NONE', #3654 ) ;
#6978=VERTEX_POINT ( 'NONE', #5659 ) ;
#6988=DIRECTION ( 'NONE',  ( -3.032184104443272185E-30, -1.000000000000000000, 7.395570986447005381E-32 ) ) ;
#7002=ORIENTED_EDGE ( 'NONE', *, *, #19177, .T. ) ;
#7010=DIRECTION ( 'NONE',  ( 3.330669073875432643E-16, 4.437342591868153746E-31, -1.000000000000000000 ) ) ;
#7011=ORIENTED_EDGE ( 'NONE', *, *, #979, .T. ) ;
#7012=DIRECTION ( 'NONE',  ( 3.330669073875432643E-16, 4.437342591868153746E-31, -1.000000000000000000 ) ) ;
#7019=DIRECTION ( 'NONE',  ( 1.000000000000000000, 2.699383410053119644E-30, 3.330669073875432643E-16 ) ) ;
#7021=CARTESIAN_POINT ( 'NONE',  ( 83.98338480886826574, -11.64708151429766403, -6.000000000000019540 ) ) ;
#7023=DIRECTION ( 'NONE',  ( -3.885780586188016830E-16, -4.437342591868156373E-31, 1.000000000000000000 ) ) ;
#7031=AXIS2_PLACEMENT_3D ( 'NONE', #6084, #13028, #11257 ) ;
#7048=AXIS2_PLACEMENT_3D ( 'NONE', #9903, #13547, #10017 ) ;
#7052=EDGE_CURVE ( 'NONE', #13332, #22506, #14574, .T. ) ;
#7055=DIRECTION ( 'NONE',  ( -3.885780586188016830E-16, -4.437342591868156373E-31, 1.000000000000000000 ) ) ;
#7071=DIRECTION ( 'NONE',  ( 3.885780586188016830E-16, 4.437342591868156373E-31, -1.000000000000000000 ) ) ;
#7072=CYLINDRICAL_SURFACE ( 'NONE', #15428, 0.5000000000000025535 ) ;
#7073=PRODUCT ( 'Half Handle', 'Half Handle', '', ( #21883 ) ) ;
#7087=CIRCLE ( 'NONE', #18335, 0.4999999999999990563 ) ;
#7094=ORIENTED_EDGE ( 'NONE', *, *, #13394, .F. ) ;
#7095=EDGE_CURVE ( 'NONE', #9218, #6497, #18701, .T. ) ;
#7113=DIRECTION ( 'NONE',  ( -1.000000000000000000, -2.699383410053119644E-30, -3.330669073875432643E-16 ) ) ;
#7115=CARTESIAN_POINT ( 'NONE',  ( 86.02937988905580369, -11.02760560296348125, -6.499999999999943157 ) ) ;
#7123=VERTEX_POINT ( 'NONE', #2344 ) ;
#7130=VERTEX_POINT ( 'NONE', #20587 ) ;
#7134=DIRECTION ( 'NONE',  ( -1.000000000000000000, -2.699383410053119644E-30, -3.330669073875432643E-16 ) ) ;
#7138=CARTESIAN_POINT ( 'NONE',  ( 110.9706201109471522, -9.453020409440265226, 6.500000000000095923 ) ) ;
#7165=FACE_OUTER_BOUND ( 'NONE', #17634, .T. ) ;
#7166=LINE ( 'NONE', #14449, #12900 ) ;
#7176=VERTEX_POINT ( 'NONE', #13404 ) ;
#7206=EDGE_CURVE ( 'NONE', #21696, #9536, #13975, .T. ) ;
#7215=FACE_OUTER_BOUND ( 'NONE', #11482, .T. ) ;
#7218=CARTESIAN_POINT ( 'NONE',  ( 114.8016533820239573, -4.500000000000059508, -6.499999999999964473 ) ) ;
#7242=EDGE_CURVE ( 'NONE', #13332, #6496, #1064, .T. ) ;
#7262=ORIENTED_EDGE ( 'NONE', *, *, #6232, .T. ) ;
#7274=FACE_OUTER_BOUND ( 'NONE', #572, .T. ) ;
#7277=DIRECTION ( 'NONE',  ( 3.885780586188016830E-16, 4.437342591868156373E-31, -1.000000000000000000 ) ) ;
#7298=CARTESIAN_POINT ( 'NONE',  ( 77.42435809754135789, -3.999999999999809042, 6.500000000000137668 ) ) ;
#7333=DIRECTION ( 'NONE',  ( 0.7313537016191735685, -0.6819983600624951459, 3.923113172947598083E-16 ) ) ;
#7336=DIRECTION ( 'NONE',  ( 1.000000000000000000, 2.699383410053119644E-30, 3.330669073875432643E-16 ) ) ;
#7343=ORIENTED_EDGE ( 'NONE', *, *, #11284, .T. ) ;
#7346=ORIENTED_EDGE ( 'NONE', *, *, #14053, .F. ) ;
#7357=FACE_OUTER_BOUND ( 'NONE', #13331, .T. ) ;
#7369=ORIENTED_EDGE ( 'NONE', *, *, #14686, .F. ) ;
#7373=ADVANCED_FACE ( 'NONE', ( #3631 ), #12561, .T. ) ;
#7380=DIRECTION ( 'NONE',  ( 0.6819983600624981435, -0.7313537016191709039, 0.000000000000000000 ) ) ;
#7384=LINE ( 'NONE', #14447, #13201 ) ;
#7390=VECTOR ( 'NONE', #5715, 1000.000000000000000 ) ;
#7398=CARTESIAN_POINT ( 'NONE',  ( 58.04599508018841192, 2.194061104857452982, 6.500000000000199840 ) ) ;
#7400=VECTOR ( 'NONE', #4556, 1000.000000000000000 ) ;
#7403=LINE ( 'NONE', #349, #11841 ) ;
#7406=CIRCLE ( 'NONE', #5154, 6.500000000000075495 ) ;
#7422=ADVANCED_FACE ( 'NONE', ( #14556 ), #17218, .T. ) ;
#7428=EDGE_LOOP ( 'NONE', ( #22265, #15582, #10143, #10120 ) ) ;
#7429=LINE ( 'NONE', #18248, #19302 ) ;
#7437=CARTESIAN_POINT ( 'NONE',  ( 119.5756419024615553, -11.00000000000006573, 6.500000000000012434 ) ) ;
#7440=CARTESIAN_POINT ( 'NONE',  ( 108.2426266706970779, -6.527605602963587828, 6.000000000000109246 ) ) ;
#7444=CIRCLE ( 'NONE', #2942, 0.5000000000000038858 ) ;
#7460=VERTEX_POINT ( 'NONE', #3288 ) ;
#7461=CARTESIAN_POINT ( 'NONE',  ( 88.75737332930594903, -6.527605602963476805, 6.500000000000151879 ) ) ;
#7470=ADVANCED_FACE ( 'NONE', ( #23051 ), #1739, .T. ) ;
#7472=DIRECTION ( 'NONE',  ( 3.241725282392603095E-30, 1.000000000000000000, -2.218671295934100958E-31 ) ) ;
#7513=PLANE ( 'NONE',  #9463 ) ;
#7521=CARTESIAN_POINT ( 'NONE',  ( 108.2426266706970637, -10.52760560296359138, 5.999999999999984901 ) ) ;
#7526=DIRECTION ( 'NONE',  ( 3.885780586188016830E-16, 4.437342591868156373E-31, -1.000000000000000000 ) ) ;
#7529=EDGE_CURVE ( 'NONE', #6413, #10566, #1828, .T. ) ;
#7530=CARTESIAN_POINT ( 'NONE',  ( 6.500000000000227374, 3.000000000000197176, 6.000000000000213163 ) ) ;
#7546=CIRCLE ( 'NONE', #1908, 0.4999999999999978351 ) ;
#7552=CARTESIAN_POINT ( 'NONE',  ( 124.5000000000017195, -4.000000000000058620, 1.387778780781445676E-14 ) ) ;
#7564=AXIS2_PLACEMENT_3D ( 'NONE', #4416, #17234, #15470 ) ;
#7569=ORIENTED_EDGE ( 'NONE', *, *, #10869, .F. ) ;
#7597=AXIS2_PLACEMENT_3D ( 'NONE', #4292, #18776, #11469 ) ;
#7601=FACE_OUTER_BOUND ( 'NONE', #18072, .T. ) ;
#7648=CIRCLE ( 'NONE', #12529, 0.5000000000000038858 ) ;
#7680=ORIENTED_EDGE ( 'NONE', *, *, #21339, .F. ) ;
#7695=ORIENTED_EDGE ( 'NONE', *, *, #1268, .F. ) ;
#7696=LINE ( 'NONE', #19938, #9548 ) ;
#7716=EDGE_CURVE ( 'NONE', #19728, #11543, #9746, .T. ) ;
#7719=ORIENTED_EDGE ( 'NONE', *, *, #18361, .T. ) ;
#7721=CARTESIAN_POINT ( 'NONE',  ( 86.00000000000117950, -10.52760560296347947, 6.000000000000054179 ) ) ;
#7735=VECTOR ( 'NONE', #20441, 1000.000000000000000 ) ;
#7739=ORIENTED_EDGE ( 'NONE', *, *, #5645, .T. ) ;
#7743=CARTESIAN_POINT ( 'NONE',  ( 108.2426266706970637, -6.527605602963671316, -5.999999999999991118 ) ) ;
#7750=LINE ( 'NONE', #13170, #12524 ) ;
#7762=ORIENTED_EDGE ( 'NONE', *, *, #11839, .T. ) ;
#7777=DIRECTION ( 'NONE',  ( -0.6819983600624998088, -0.7313537016191693496, 0.000000000000000000 ) ) ;
#7790=AXIS2_PLACEMENT_3D ( 'NONE', #13348, #13577, #20530 ) ;
#7801=ADVANCED_FACE ( 'NONE', ( #3712 ), #19726, .T. ) ;
#7804=ORIENTED_EDGE ( 'NONE', *, *, #4874, .T. ) ;
#7805=EDGE_CURVE ( 'NONE', #12275, #6044, #11980, .T. ) ;
#7807=CARTESIAN_POINT ( 'NONE',  ( 77.42435809754137210, -6.999999999999811706, 6.500000000000081712 ) ) ;
#7810=DIRECTION ( 'NONE',  ( 3.885780586188016830E-16, 4.437342591868156373E-31, -1.000000000000000000 ) ) ;
#7824=ORIENTED_EDGE ( 'NONE', *, *, #12263, .F. ) ;
#7834=DIRECTION ( 'NONE',  ( -0.7313537016191756779, 0.6819983600624930364, -4.000536147326505450E-15 ) ) ;
#7841=ADVANCED_FACE ( 'NONE', ( #12293 ), #19484, .T. ) ;
#7843=FACE_OUTER_BOUND ( 'NONE', #4680, .T. ) ;
#7849=EDGE_CURVE ( 'NONE', #19782, #273, #17613, .T. ) ;
#7865=CARTESIAN_POINT ( 'NONE',  ( 66.26395429947837101, 0.000000000000000000, -5.999999999999908518 ) ) ;
#7868=DIRECTION ( 'NONE',  ( -3.885780586188016830E-16, -4.437342591868156373E-31, 1.000000000000000000 ) ) ;
#7869=ADVANCED_FACE ( 'NONE', ( #5949 ), #2977, .T. ) ;
#7880=VERTEX_POINT ( 'NONE', #13006 ) ;
#7891=CARTESIAN_POINT ( 'NONE',  ( 2.498001805406602216E-13, 2.500000000000002220, 6.000000000000158096 ) ) ;
#7895=CARTESIAN_POINT ( 'NONE',  ( 78.36587326203827786, -2.990348597579628454, -5.999999999999998224 ) ) ;
#7903=CARTESIAN_POINT ( 'NONE',  ( 63.50658097017376491, -4.000000000000058620, -6.000000000000054179 ) ) ;
#7909=ADVANCED_FACE ( 'NONE', ( #2174 ), #9362, .T. ) ;
#7918=FACE_OUTER_BOUND ( 'NONE', #2853, .T. ) ;
#7920=FACE_OUTER_BOUND ( 'NONE', #9644, .T. ) ;
#7928=LINE ( 'NONE', #20646, #16428 ) ;
#7929=CARTESIAN_POINT ( 'NONE',  ( 82.19834661797897013, -5.880524088665628923, 6.500000000000151879 ) ) ;
#7962=SURFACE_STYLE_USAGE ( .BOTH. , #683 ) ;
#7979=DIRECTION ( 'NONE',  ( 3.885780586188016830E-16, 4.437342591868156373E-31, -1.000000000000000000 ) ) ;
#7988=DIRECTION ( 'NONE',  ( 0.000000000000000000, 0.000000000000000000, 1.000000000000000000 ) ) ;
#7992=CYLINDRICAL_SURFACE ( 'NONE', #3249, 2.550000000000012701 ) ;
#8000=AXIS2_PLACEMENT_3D ( 'NONE', #15925, #1709, #15804 ) ;
#8001=CIRCLE ( 'NONE', #15513, 6.500000000000052403 ) ;
#8008=ORIENTED_EDGE ( 'NONE', *, *, #17314, .F. ) ;
#8016=AXIS2_PLACEMENT_3D ( 'NONE', #8734, #6988, #14146 ) ;
#8027=ORIENTED_EDGE ( 'NONE', *, *, #1892, .F. ) ;
#8039=CARTESIAN_POINT ( 'NONE',  ( 66.26395429947839943, -7.000000000000006217, -6.499999999999999112 ) ) ;
#8047=CARTESIAN_POINT ( 'NONE',  ( 66.26395429947837101, -4.500000000000003553, 6.500000000000110134 ) ) ;
#8049=FACE_OUTER_BOUND ( 'NONE', #740, .T. ) ;
#8059=ADVANCED_FACE ( 'NONE', ( #5561 ), #11609, .T. ) ;
#8072=EDGE_CURVE ( 'NONE', #10144, #14358, #15372, .T. ) ;
#8073=DIRECTION ( 'NONE',  ( 2.242473278838646163E-61, 7.395570986447005381E-32, 1.000000000000000000 ) ) ;
#8090=EDGE_LOOP ( 'NONE', ( #21326, #704, #17182, #22796 ) ) ;
#8093=DIRECTION ( 'NONE',  ( -0.6819983600624981435, -0.7313537016191709039, 0.000000000000000000 ) ) ;
#8094=EDGE_CURVE ( 'NONE', #13307, #20921, #4474, .T. ) ;
#8106=LINE ( 'NONE', #19157, #20812 ) ;
#8109=FACE_OUTER_BOUND ( 'NONE', #21413, .T. ) ;
#8114=EDGE_CURVE ( 'NONE', #19862, #10112, #1244, .T. ) ;
#8135=DIRECTION ( 'NONE',  ( -1.000000000000000000, 0.000000000000000000, -2.668805347656595124E-16 ) ) ;
#8149=ORIENTED_EDGE ( 'NONE', *, *, #8094, .T. ) ;
#8160=FACE_OUTER_BOUND ( 'NONE', #5469, .T. ) ;
#8183=TOROIDAL_SURFACE ( 'NONE', #10060, 6.500000000000000888, 0.5000000000000000000 ) ;
#8192=FACE_OUTER_BOUND ( 'NONE', #18564, .T. ) ;
#8194=AXIS2_PLACEMENT_3D ( 'NONE', #3107, #1799, #21106 ) ;
#8196=DIRECTION ( 'NONE',  ( 1.000000000000000000, 5.598259082250514647E-17, 3.330669073875432643E-16 ) ) ;
#8212=CARTESIAN_POINT ( 'NONE',  ( 61.83096495907210510, -4.753799060524588782, 6.000000000000123457 ) ) ;
#8233=AXIS2_PLACEMENT_3D ( 'NONE', #15938, #15710, #16052 ) ;
#8245=LINE ( 'NONE', #8354, #13818 ) ;
#8248=CARTESIAN_POINT ( 'NONE',  ( 6.500000000000283329, 0.5000000000001669775, -5.999999999999943157 ) ) ;
#8254=FACE_OUTER_BOUND ( 'NONE', #12034, .T. ) ;
#8279=FACE_OUTER_BOUND ( 'NONE', #1701, .T. ) ;
#8291=ORIENTED_EDGE ( 'NONE', *, *, #8952, .F. ) ;
#8293=VERTEX_POINT ( 'NONE', #22683 ) ;
#8294=ADVANCED_FACE ( 'NONE', ( #9978 ), #6570, .F. ) ;
#8303=ADVANCED_FACE ( 'NONE', ( #3389 ), #18168, .F. ) ;
#8306=CARTESIAN_POINT ( 'NONE',  ( 54.42435809754109499, 0.000000000000000000, 6.500000000000144773 ) ) ;
#8308=CARTESIAN_POINT ( 'NONE',  ( 86.00000000000137845, -13.52760560296348302, 6.500000000000117240 ) ) ;
#8313=ORIENTED_EDGE ( 'NONE', *, *, #15592, .F. ) ;
#8320=VERTEX_POINT ( 'NONE', #14630 ) ;
#8330=CARTESIAN_POINT ( 'NONE',  ( 116.5066492821803052, -7.708908342713760575, 6.000000000000102141 ) ) ;
#8332=DIRECTION ( 'NONE',  ( 3.032184104443272185E-30, 1.000000000000000000, -7.395570986447005381E-32 ) ) ;
#8334=AXIS2_PLACEMENT_3D ( 'NONE', #9608, #22423, #18655 ) ;
#8346=AXIS2_PLACEMENT_3D ( 'NONE', #9482, #13485, #16985 ) ;
#8350=CARTESIAN_POINT ( 'NONE',  ( 82.19834661797897013, -5.880524088665628923, 6.500000000000151879 ) ) ;
#8354=CARTESIAN_POINT ( 'NONE',  ( 118.0000000000018190, -4.000000000000003553, 6.000000000000109246 ) ) ;
#8367=VECTOR ( 'NONE', #3591, 1000.000000000000000 ) ;
#8376=VERTEX_POINT ( 'NONE', #10436 ) ;
#8390=AXIS2_PLACEMENT_3D ( 'NONE', #9830, #22187, #15348 ) ;
#8396=CIRCLE ( 'NONE', #15895, 0.5000000000000038858 ) ;
#8397=EDGE_CURVE ( 'NONE', #7880, #13843, #179, .T. ) ;
#8403=CARTESIAN_POINT ( 'NONE',  ( 54.42435809754113052, -4.000000000000003553, -6.499999999999999112 ) ) ;
#8406=DIRECTION ( 'NONE',  ( -1.000000000000000000, 0.000000000000000000, -4.336808689941968432E-16 ) ) ;
#8410=VECTOR ( 'NONE', #10561, 1000.000000000000000 ) ;
#8416=AXIS2_PLACEMENT_3D ( 'NONE', #7865, #18452, #4319 ) ;
#8418=AXIS2_PLACEMENT_3D ( 'NONE', #4337, #12831, #720 ) ;
#8422=DIRECTION ( 'NONE',  ( 3.885780586188016830E-16, 4.437342591868156373E-31, -1.000000000000000000 ) ) ;
#8425=LINE ( 'NONE', #22540, #13145 ) ;
#8428=DIRECTION ( 'NONE',  ( 3.885780586188016830E-16, 4.437342591868156373E-31, -1.000000000000000000 ) ) ;
#8430=DIRECTION ( 'NONE',  ( 0.6819983600624998088, -0.7313537016191693496, 0.000000000000000000 ) ) ;
#8434=CARTESIAN_POINT ( 'NONE',  ( 63.50658097017375070, -4.000000000000003553, 6.000000000000185629 ) ) ;
#8475=DIRECTION ( 'NONE',  ( -0.7313537016191730133, 0.6819983600624958120, -5.924440990721418971E-17 ) ) ;
#8477=DIRECTION ( 'NONE',  ( -1.000000000000000000, -2.699383410053119644E-30, -3.330669073875432643E-16 ) ) ;
#8480=DIRECTION ( 'NONE',  ( 0.000000000000000000, 0.000000000000000000, 1.000000000000000000 ) ) ;
#8485=DIRECTION ( 'NONE',  ( 3.885780586188016830E-16, 4.437342591868156373E-31, -1.000000000000000000 ) ) ;
#8495=ORIENTED_EDGE ( 'NONE', *, *, #1118, .T. ) ;
#8517=VERTEX_POINT ( 'NONE', #4143 ) ;
#8522=VECTOR ( 'NONE', #8563, 1000.000000000000000 ) ;
#8525=VECTOR ( 'NONE', #16024, 1000.000000000000000 ) ;
#8528=CARTESIAN_POINT ( 'NONE',  ( 119.5756419024616690, -7.000000000000062172, -6.500000000000033751 ) ) ;
#8529=EDGE_CURVE ( 'NONE', #13843, #5583, #21816, .T. ) ;
#8532=EDGE_CURVE ( 'NONE', #15636, #6497, #21932, .T. ) ;
#8535=CARTESIAN_POINT ( 'NONE',  ( 84.32438398889958364, -11.28140466348809312, -6.500000000000026645 ) ) ;
#8537=DIRECTION ( 'NONE',  ( 0.000000000000000000, 0.000000000000000000, 1.000000000000000000 ) ) ;
#8549=LINE ( 'NONE', #19486, #8564 ) ;
#8552=AXIS2_PLACEMENT_3D ( 'NONE', #5569, #14383, #12380 ) ;
#8554=ORIENTED_EDGE ( 'NONE', *, *, #17222, .T. ) ;
#8559=DIRECTION ( 'NONE',  ( 1.000000000000000000, 2.699383410053119644E-30, 3.330669073875432643E-16 ) ) ;
#8562=EDGE_CURVE ( 'NONE', #4606, #3634, #3143, .T. ) ;
#8563=DIRECTION ( 'NONE',  ( 1.000000000000000000, 5.598259082250514647E-17, 3.330669073875432643E-16 ) ) ;
#8564=VECTOR ( 'NONE', #15712, 1000.000000000000114 ) ;
#8567=CIRCLE ( 'NONE', #8935, 4.000000000000045297 ) ;
#8580=VERTEX_POINT ( 'NONE', #16602 ) ;
#8583=CIRCLE ( 'NONE', #21001, 0.4999999999999990563 ) ;
#8595=DIRECTION ( 'NONE',  ( -0.7313537016191756779, 0.6819983600624930364, 2.105690488111832645E-15 ) ) ;
#8596=DIRECTION ( 'NONE',  ( 1.000000000000000000, -1.847414967615758933E-47, 3.885780586188017323E-16 ) ) ;
#8611=FACE_OUTER_BOUND ( 'NONE', #21752, .T. ) ;
#8616=LINE ( 'NONE', #6851, #3965 ) ;
#8633=ORIENTED_EDGE ( 'NONE', *, *, #14775, .T. ) ;
#8637=VECTOR ( 'NONE', #7810, 1000.000000000000000 ) ;
#8652=EDGE_CURVE ( 'NONE', #5256, #17475, #504, .T. ) ;
#8655=TOROIDAL_SURFACE ( 'NONE', #16162, 6.500000000000000888, 0.5000000000000000000 ) ;
#8657=CARTESIAN_POINT ( 'NONE',  ( 63.50658097017376491, -6.500000000000061284, -6.000000000000054179 ) ) ;
#8662=PLANE ( 'NONE',  #22467 ) ;
#8667=ORIENTED_EDGE ( 'NONE', *, *, #21500, .F. ) ;
#8684=ADVANCED_FACE ( 'NONE', ( #4608 ), #20973, .T. ) ;
#8719=AXIS2_PLACEMENT_3D ( 'NONE', #1389, #3161, #4793 ) ;
#8723=EDGE_CURVE ( 'NONE', #10112, #4169, #22673, .T. ) ;
#8727=CARTESIAN_POINT ( 'NONE',  ( 6.500000000000227374, 2.500000000000141220, 4.163336342344337027E-14 ) ) ;
#8728=CARTESIAN_POINT ( 'NONE',  ( 77.42435809754135789, -6.499999999999811706, 6.500000000000137668 ) ) ;
#8733=DIRECTION ( 'NONE',  ( -1.000000000000000000, -2.699383410053119644E-30, -3.330669073875432643E-16 ) ) ;
#8734=CARTESIAN_POINT ( 'NONE',  ( 124.5000000000019469, -7.000000000000062172, 2.081668171172168513E-14 ) ) ;
#8746=DIRECTION ( 'NONE',  ( 3.885780586188016830E-16, 4.437342591868156373E-31, -1.000000000000000000 ) ) ;
#8784=DIRECTION ( 'NONE',  ( -3.885780586188016830E-16, -4.437342591868156373E-31, 1.000000000000000000 ) ) ;
#8790=EDGE_CURVE ( 'NONE', #14827, #5349, #8001, .T. ) ;
#8791=DIRECTION ( 'NONE',  ( 0.000000000000000000, 0.000000000000000000, 1.000000000000000000 ) ) ;
#8794=DIRECTION ( 'NONE',  ( -0.6819983600624998088, -0.7313537016191693496, 0.000000000000000000 ) ) ;
#8803=DIRECTION ( 'NONE',  ( 1.000000000000000000, 2.699383410053119644E-30, 3.330669073875432643E-16 ) ) ;
#8816=EDGE_LOOP ( 'NONE', ( #13896, #10749, #14162, #15595 ) ) ;
#8828=CARTESIAN_POINT ( 'NONE',  ( 108.2426266706970353, -6.527605602963587828, 6.500000000000199840 ) ) ;
#8836=PLANE ( 'NONE',  #18343 ) ;
#8841=ORIENTED_EDGE ( 'NONE', *, *, #18293, .T. ) ;
#8855=EDGE_CURVE ( 'NONE', #22680, #16775, #6142, .T. ) ;
#8860=DIRECTION ( 'NONE',  ( -0.6819983600624989206, -0.7313537016191700157, 0.000000000000000000 ) ) ;
#8883=CARTESIAN_POINT ( 'NONE',  ( 80.15235153779143218, -8.074585193523137860, -6.000000000000060396 ) ) ;
#8891=LINE ( 'NONE', #7021, #17997 ) ;
#8897=CARTESIAN_POINT ( 'NONE',  ( 77.42435809754145737, -3.999999999999809042, -6.499999999999984901 ) ) ;
#8901=AXIS2_PLACEMENT_3D ( 'NONE', #15815, #7023, #17838 ) ;
#8908=LINE ( 'NONE', #1611, #13665 ) ;
#8909=CARTESIAN_POINT ( 'NONE',  ( 116.8476484622116232, -8.074585193523331483, 6.500000000000040856 ) ) ;
#8912=CARTESIAN_POINT ( 'NONE',  ( 66.26395429947831417, -4.000000000000003553, 6.000000000000192735 ) ) ;
#8924=CIRCLE ( 'NONE', #4022, 2.550000000000024691 ) ;
#8928=ADVANCED_FACE ( 'NONE', ( #13304 ), #5671, .T. ) ;
#8935=AXIS2_PLACEMENT_3D ( 'NONE', #21765, #125, #15862 ) ;
#8940=CARTESIAN_POINT ( 'NONE',  ( 54.42435809754115894, 2.999999999999947153, -5.999999999999950262 ) ) ;
#8943=CARTESIAN_POINT ( 'NONE',  ( 114.8016533820240426, -5.880524088665822546, 6.500000000000123457 ) ) ;
#8952=EDGE_CURVE ( 'NONE', #4310, #14732, #7429, .T. ) ;
#8978=VECTOR ( 'NONE', #23007, 1000.000000000000000 ) ;
#8981=EDGE_CURVE ( 'NONE', #19728, #19565, #22238, .T. ) ;
#8984=LINE ( 'NONE', #7115, #19837 ) ;
#8988=VERTEX_POINT ( 'NONE', #11757 ) ;
#8990=EDGE_CURVE ( 'NONE', #14077, #4310, #6245, .T. ) ;
#9000=CARTESIAN_POINT ( 'NONE',  ( 66.26395429947837101, -4.000000000000003553, 6.500000000000110134 ) ) ;
#9001=AXIS2_PLACEMENT_3D ( 'NONE', #21537, #351, #234 ) ;
#9005=CARTESIAN_POINT ( 'NONE',  ( 88.75737332930592061, -6.527605602963476805, -6.000000000000012434 ) ) ;
#9012=EDGE_LOOP ( 'NONE', ( #22306, #14757, #4463, #4815 ) ) ;
#9013=DIRECTION ( 'NONE',  ( 1.000000000000000000, 1.503427012513217564E-14, 3.854941057726199147E-16 ) ) ;
#9016=ORIENTED_EDGE ( 'NONE', *, *, #20482, .T. ) ;
#9022=ADVANCED_FACE ( 'NONE', ( #6469 ), #10004, .T. ) ;
#9032=CARTESIAN_POINT ( 'NONE',  ( 77.42435809754137210, -4.499999999999809930, -5.999999999999984901 ) ) ;
#9046=CARTESIAN_POINT ( 'NONE',  ( 83.98338480886823731, -11.64708151429766403, 6.500000000000117240 ) ) ;
#9055=DIRECTION ( 'NONE',  ( 0.000000000000000000, 0.000000000000000000, -1.000000000000000000 ) ) ;
#9087=PLANE ( 'NONE',  #16799 ) ;
#9096=ORIENTED_EDGE ( 'NONE', *, *, #5182, .T. ) ;
#9110=VECTOR ( 'NONE', #21152, 1000.000000000000000 ) ;
#9133=VECTOR ( 'NONE', #5141, 1000.000000000000000 ) ;
#9140=DIRECTION ( 'NONE',  ( -1.000000000000000000, 0.000000000000000000, -4.336808689941968432E-16 ) ) ;
#9148=AXIS2_PLACEMENT_3D ( 'NONE', #5217, #17803, #15898 ) ;
#9154=DIRECTION ( 'NONE',  ( 3.330669073875432643E-16, 4.437342591868153746E-31, -1.000000000000000000 ) ) ;
#9165=AXIS2_PLACEMENT_3D ( 'NONE', #315, #2416, #9252 ) ;
#9167=DIRECTION ( 'NONE',  ( 0.6819983600624971443, -0.7313537016191717921, 0.000000000000000000 ) ) ;
#9181=DIRECTION ( 'NONE',  ( -3.330669073875432643E-16, -4.437342591868153746E-31, 1.000000000000000000 ) ) ;
#9186=ORIENTED_EDGE ( 'NONE', *, *, #18748, .T. ) ;
#9213=ORIENTED_EDGE ( 'NONE', *, *, #2640, .T. ) ;
#9218=VERTEX_POINT ( 'NONE', #6946 ) ;
#9226=EDGE_CURVE ( 'NONE', #8320, #15636, #13988, .T. ) ;
#9229=DIRECTION ( 'NONE',  ( -1.000000000000000000, -2.699383410053119293E-30, -4.336808689941968432E-16 ) ) ;
#9230=EDGE_CURVE ( 'NONE', #2822, #9536, #7648, .T. ) ;
#9237=DIRECTION ( 'NONE',  ( -1.000000000000000000, -2.699383410053120695E-30, -3.885780586188017323E-16 ) ) ;
#9242=DIRECTION ( 'NONE',  ( 1.000000000000000000, 2.699383410053119644E-30, 3.330669073875432643E-16 ) ) ;
#9243=ORIENTED_EDGE ( 'NONE', *, *, #21410, .T. ) ;
#9252=DIRECTION ( 'NONE',  ( -0.6819983600625070252, -0.7313537016191624662, 0.000000000000000000 ) ) ;
#9266=DIRECTION ( 'NONE',  ( -1.000000000000000000, 0.000000000000000000, -4.336808689941968432E-16 ) ) ;
#9272=ORIENTED_EDGE ( 'NONE', *, *, #21914, .F. ) ;
#9293=DIRECTION ( 'NONE',  ( -0.7313537016191733464, 0.6819983600624954789, -3.733258675956565293E-18 ) ) ;
#9294=DIRECTION ( 'NONE',  ( 3.241725282392603095E-30, 1.000000000000000000, -2.218671295934100958E-31 ) ) ;
#9301=EDGE_CURVE ( 'NONE', #6421, #18645, #16649, .T. ) ;
#9307=EDGE_CURVE ( 'NONE', #14358, #14050, #20225, .T. ) ;
#9314=AXIS2_PLACEMENT_3D ( 'NONE', #4388, #4515, #15090 ) ;
#9325=VECTOR ( 'NONE', #4104, 1000.000000000000000 ) ;
#9326=DIRECTION ( 'NONE',  ( -0.6819983600624940356, 0.7313537016191746787, 1.110361430785838977E-16 ) ) ;
#9335=EDGE_LOOP ( 'NONE', ( #22211, #1610, #16399, #2464 ) ) ;
#9344=AXIS2_PLACEMENT_3D ( 'NONE', #2889, #22312, #20899 ) ;
#9346=CARTESIAN_POINT ( 'NONE',  ( 58.85734743794747459, 0.7537990605245292741, 6.000000000000158096 ) ) ;
#9351=CARTESIAN_POINT ( 'NONE',  ( 110.9706201109471522, -9.453020409440265226, 6.500000000000095923 ) ) ;
#9354=EDGE_CURVE ( 'NONE', #12275, #10139, #13161, .T. ) ;
#9362=CYLINDRICAL_SURFACE ( 'NONE', #21776, 6.500000000000052403 ) ;
#9371=DIRECTION ( 'NONE',  ( 1.000000000000000000, 2.699383410053119644E-30, 3.330669073875432643E-16 ) ) ;
#9373=DIRECTION ( 'NONE',  ( -4.003208021484906984E-16, 0.000000000000000000, 1.000000000000000000 ) ) ;
#9381=DIRECTION ( 'NONE',  ( -0.6819983600625060260, -0.7313537016191635765, -6.106365041599011361E-16 ) ) ;
#9384=DIRECTION ( 'NONE',  ( 3.032184104443272185E-30, 1.000000000000000000, -7.395570986447005381E-32 ) ) ;
#9387=SURFACE_STYLE_FILL_AREA ( #797 ) ;
#9403=CARTESIAN_POINT ( 'NONE',  ( 108.2426266706971205, -10.52760560296367487, -6.500000000000075495 ) ) ;
#9406=EDGE_CURVE ( 'NONE', #18021, #16591, #20376, .T. ) ;
#9414=DIRECTION ( 'NONE',  ( -0.7313537016191746787, -0.6819983600624941467, -1.072890437865584409E-16 ) ) ;
#9419=CIRCLE ( 'NONE', #15777, 2.550000000000012701 ) ;
#9421=VERTEX_POINT ( 'NONE', #18675 ) ;
#9426=DIRECTION ( 'NONE',  ( -1.000000000000000000, -2.699383410053119644E-30, -3.330669073875432643E-16 ) ) ;
#9427=ORIENTED_EDGE ( 'NONE', *, *, #21471, .F. ) ;
#9437=SURFACE_SIDE_STYLE ('',( #4352 ) ) ;
#9449=ORIENTED_EDGE ( 'NONE', *, *, #12716, .T. ) ;
#9455=ORIENTED_EDGE ( 'NONE', *, *, #9638, .F. ) ;
#9459=DIRECTION ( 'NONE',  ( 3.032184104443272185E-30, 1.000000000000000000, -7.395570986447005381E-32 ) ) ;
#9461=CARTESIAN_POINT ( 'NONE',  ( 63.53596085922838199, -2.925414806476733798, -6.000000000000060396 ) ) ;
#9463=AXIS2_PLACEMENT_3D ( 'NONE', #7398, #22095, #19869 ) ;
#9470=VERTEX_POINT ( 'NONE', #22446 ) ;
#9482=CARTESIAN_POINT ( 'NONE',  ( 88.75737332930596324, -6.527605602963476805, 6.000000000000165201 ) ) ;
#9507=DIRECTION ( 'NONE',  ( 1.000000000000000000, 1.871023177660678976E-14, 3.717264591378832268E-16 ) ) ;
#9519=EDGE_CURVE ( 'NONE', #21618, #21696, #1604, .T. ) ;
#9520=DIRECTION ( 'NONE',  ( -0.6819983600624998088, 0.7313537016191693496, 0.000000000000000000 ) ) ;
#9523=FACE_OUTER_BOUND ( 'NONE', #2273, .T. ) ;
#9536=VERTEX_POINT ( 'NONE', #11853 ) ;
#9544=ORIENTED_EDGE ( 'NONE', *, *, #21914, .T. ) ;
#9548=VECTOR ( 'NONE', #2042, 1000.000000000000000 ) ;
#9563=CIRCLE ( 'NONE', #12563, 7.000000000000075495 ) ;
#9581=AXIS2_PLACEMENT_3D ( 'NONE', #13076, #20135, #2252 ) ;
#9591=CARTESIAN_POINT ( 'NONE',  ( 6.500000000000172307, -13.52760560296348302, -2.081668171172168513E-14 ) ) ;
#9608=CARTESIAN_POINT ( 'NONE',  ( 81.04599508018871745, -4.805938895142302769, 6.500000000000144773 ) ) ;
#9610=DIRECTION ( 'NONE',  ( -1.000000000000000000, 0.000000000000000000, -3.717264591378832268E-16 ) ) ;
#9618=ORIENTED_EDGE ( 'NONE', *, *, #8072, .T. ) ;
#9630=DIRECTION ( 'NONE',  ( 3.330669073875432643E-16, 4.437342591868153746E-31, -1.000000000000000000 ) ) ;
#9636=CYLINDRICAL_SURFACE ( 'NONE', #10464, 2.550000000000012701 ) ;
#9638=EDGE_CURVE ( 'NONE', #9218, #19862, #10438, .T. ) ;
#9644=EDGE_LOOP ( 'NONE', ( #2610, #17656, #21610, #7739 ) ) ;
#9653=DIRECTION ( 'NONE',  ( 3.241725282392603095E-30, 1.000000000000000000, -2.218671295934100958E-31 ) ) ;
#9663=ADVANCED_FACE ( 'NONE', ( #3496 ), #17723, .T. ) ;
#9665=FACE_OUTER_BOUND ( 'NONE', #19593, .T. ) ;
#9690=LINE ( 'NONE', #10151, #8637 ) ;
#9712=ORIENTED_EDGE ( 'NONE', *, *, #10549, .F. ) ;
#9734=PRESENTATION_STYLE_ASSIGNMENT (( #7962 ) ) ;
#9737=VERTEX_POINT ( 'NONE', #18310 ) ;
#9741=ORIENTED_EDGE ( 'NONE', *, *, #20596, .T. ) ;
#9743=VERTEX_POINT ( 'NONE', #13135 ) ;
#9746=CIRCLE ( 'NONE', #8233, 0.5000000000000038858 ) ;
#9748=ORIENTED_EDGE ( 'NONE', *, *, #6520, .F. ) ;
#9759=CARTESIAN_POINT ( 'NONE',  ( 119.5756419024615269, -4.000000000000003553, 6.500000000000123457 ) ) ;
#9764=ORIENTED_EDGE ( 'NONE', *, *, #6786, .F. ) ;
#9779=SURFACE_STYLE_USAGE ( .BOTH. , #9437 ) ;
#9796=CARTESIAN_POINT ( 'NONE',  ( 85.68838070902461368, -9.818697260249752645, -6.000000000000032863 ) ) ;
#9797=DIRECTION ( 'NONE',  ( -1.000000000000000000, -2.699383410053119644E-30, -3.330669073875432643E-16 ) ) ;
#9809=EDGE_CURVE ( 'NONE', #8293, #6413, #13632, .T. ) ;
#9830=CARTESIAN_POINT ( 'NONE',  ( 80.49335071782266482, -7.708908342713538531, 6.000000000000081712 ) ) ;
#9832=ORIENTED_EDGE ( 'NONE', *, *, #7095, .T. ) ;
#9848=AXIS2_PLACEMENT_3D ( 'NONE', #14803, #5874, #18678 ) ;
#9850=EDGE_LOOP ( 'NONE', ( #2792, #10337, #13597, #13477 ) ) ;
#9857=ORIENTED_EDGE ( 'NONE', *, *, #2209, .F. ) ;
#9860=EDGE_CURVE ( 'NONE', #12089, #20860, #12510, .T. ) ;
#9861=CARTESIAN_POINT ( 'NONE',  ( 84.32438398889955522, -11.28140466348809312, -5.999999999999956479 ) ) ;
#9868=CIRCLE ( 'NONE', #16978, 7.000000000000075495 ) ;
#9879=ORIENTED_EDGE ( 'NONE', *, *, #2261, .F. ) ;
#9891=CARTESIAN_POINT ( 'NONE',  ( 59.19834661797869302, 0.4999999999999449329, 6.000000000000165201 ) ) ;
#9903=CARTESIAN_POINT ( 'NONE',  ( 63.19496167919713514, -3.291091657286332683, -5.999999999999998224 ) ) ;
#9918=AXIS2_PLACEMENT_3D ( 'NONE', #17917, #16362, #8860 ) ;
#9925=LINE ( 'NONE', #868, #18295 ) ;
#9935=AXIS2_PLACEMENT_3D ( 'NONE', #16933, #16581, #15181 ) ;
#9945=ORIENTED_EDGE ( 'NONE', *, *, #21471, .T. ) ;
#9946=EDGE_CURVE ( 'NONE', #16059, #1495, #14766, .T. ) ;
#9960=CARTESIAN_POINT ( 'NONE',  ( 80.15235153779141797, -8.074585193523137860, -6.500000000000019540 ) ) ;
#9976=EDGE_LOOP ( 'NONE', ( #17125, #11632, #11688, #9272 ) ) ;
#9978=FACE_OUTER_BOUND ( 'NONE', #2386, .T. ) ;
#9988=DIRECTION ( 'NONE',  ( 0.000000000000000000, 0.000000000000000000, 1.000000000000000000 ) ) ;
#9994=PLANE ( 'NONE',  #15887 ) ;
#9998=EDGE_LOOP ( 'NONE', ( #10489, #12127, #18698, #10710 ) ) ;
#10004=PLANE ( 'NONE',  #5027 ) ;
#10011=DIRECTION ( 'NONE',  ( 0.000000000000000000, 0.000000000000000000, 1.000000000000000000 ) ) ;
#10017=DIRECTION ( 'NONE',  ( -0.6819983600624989206, -0.7313537016191700157, 0.000000000000000000 ) ) ;
#10019=AXIS2_PLACEMENT_3D ( 'NONE', #19735, #22920, #14085 ) ;
#10020=CYLINDRICAL_SURFACE ( 'NONE', #11564, 0.4999999999999978351 ) ;
#10022=CARTESIAN_POINT ( 'NONE',  ( 54.42435809754118736, 2.499999999999946709, -6.499999999999922728 ) ) ;
#10034=AXIS2_PLACEMENT_3D ( 'NONE', #7807, #22160, #15077 ) ;
#10054=AXIS2_PLACEMENT_3D ( 'NONE', #12415, #8784, #14075 ) ;
#10060=AXIS2_PLACEMENT_3D ( 'NONE', #14275, #21688, #18263 ) ;
#10085=VECTOR ( 'NONE', #10177, 1000.000000000000000 ) ;
#10097=ADVANCED_FACE ( 'NONE', ( #15919 ), #23128, .T. ) ;
#10098=AXIS2_PLACEMENT_3D ( 'NONE', #17868, #10563, #17741 ) ;
#10104=FACE_OUTER_BOUND ( 'NONE', #14884, .T. ) ;
#10112=VERTEX_POINT ( 'NONE', #12161 ) ;
#10120=ORIENTED_EDGE ( 'NONE', *, *, #18293, .F. ) ;
#10139=VERTEX_POINT ( 'NONE', #12753 ) ;
#10143=ORIENTED_EDGE ( 'NONE', *, *, #15233, .F. ) ;
#10144=VERTEX_POINT ( 'NONE', #12631 ) ;
#10151=CARTESIAN_POINT ( 'NONE',  ( 61.48996577904083694, -5.119475911334187224, 6.500000000000130562 ) ) ;
#10153=LINE ( 'NONE', #15437, #18948 ) ;
#10160=CARTESIAN_POINT ( 'NONE',  ( 66.26395429947841365, -7.000000000000006217, 6.500000000000075495 ) ) ;
#10164=AXIS2_PLACEMENT_3D ( 'NONE', #14145, #8733, #6852 ) ;
#10177=DIRECTION ( 'NONE',  ( 3.885780586188016830E-16, 4.437342591868156373E-31, -1.000000000000000000 ) ) ;
#10179=DIRECTION ( 'NONE',  ( -1.000000000000000000, 7.477632011778292156E-48, -3.885780586188017323E-16 ) ) ;
#10180=CARTESIAN_POINT ( 'NONE',  ( 57.49335071782236639, -0.7089083427137543580, -5.999999999999887201 ) ) ;
#10196=CYLINDRICAL_SURFACE ( 'NONE', #18192, 0.5000000000000038858 ) ;
#10201=LINE ( 'NONE', #20694, #6161 ) ;
#10212=CARTESIAN_POINT ( 'NONE',  ( 6.500000000000283329, 3.000000000000141220, -5.999999999999943157 ) ) ;
#10216=VERTEX_POINT ( 'NONE', #2155 ) ;
#10224=VECTOR ( 'NONE', #12549, 1000.000000000000114 ) ;
#10233=CARTESIAN_POINT ( 'NONE',  ( 119.5756419024615269, -4.000000000000003553, 6.500000000000123457 ) ) ;
#10297=DIRECTION ( 'NONE',  ( 3.330669073875432643E-16, 4.437342591868153746E-31, -1.000000000000000000 ) ) ;
#10301=LINE ( 'NONE', #8434, #15729 ) ;
#10316=ORIENTED_EDGE ( 'NONE', *, *, #13713, .F. ) ;
#10318=CARTESIAN_POINT ( 'NONE',  ( 2.775557561562891351E-14, 0.4999999999999726885, -6.000000000000019540 ) ) ;
#10319=DIRECTION ( 'NONE',  ( -0.7313537016191734574, 0.6819983600624954789, -3.733258675956565293E-18 ) ) ;
#10323=DIRECTION ( 'NONE',  ( -0.7313537016191746787, -0.6819983600624940356, -1.072890437865584409E-16 ) ) ;
#10337=ORIENTED_EDGE ( 'NONE', *, *, #22725, .T. ) ;
#10341=EDGE_LOOP ( 'NONE', ( #13065, #20772, #15068, #9449 ) ) ;
#10342=DIRECTION ( 'NONE',  ( 3.032184104443271834E-30, 1.000000000000000000, 4.437342591868167759E-31 ) ) ;
#10368=ORIENTED_EDGE ( 'NONE', *, *, #2484, .T. ) ;
#10372=PLANE ( 'NONE',  #20051 ) ;
#10374=AXIS2_PLACEMENT_3D ( 'NONE', #9032, #16186, #102 ) ;
#10387=EDGE_CURVE ( 'NONE', #23176, #18843, #3875, .T. ) ;
#10388=AXIS2_PLACEMENT_3D ( 'NONE', #12967, #12733, #21913 ) ;
#10395=CIRCLE ( 'NONE', #10019, 2.550000000000024691 ) ;
#10424=AXIS2_PLACEMENT_3D ( 'NONE', #11602, #6666, #18790 ) ;
#10436=CARTESIAN_POINT ( 'NONE',  ( 77.42435809754137210, -3.999999999999809042, -5.999999999999984901 ) ) ;
#10438=LINE ( 'NONE', #8909, #9110 ) ;
#10441=CARTESIAN_POINT ( 'NONE',  ( 124.5000000000017764, -4.000000000000003553, 6.000000000000116351 ) ) ;
#10442=CARTESIAN_POINT ( 'NONE',  ( 77.42435809754130105, -10.99999999999981526, 6.000000000000123457 ) ) ;
#10456=EDGE_LOOP ( 'NONE', ( #12204, #10368, #18360, #5414 ) ) ;
#10464=AXIS2_PLACEMENT_3D ( 'NONE', #11280, #16561, #14585 ) ;
#10476=DIRECTION ( 'NONE',  ( -1.000000000000000000, 0.000000000000000000, -2.668805347656595124E-16 ) ) ;
#10489=ORIENTED_EDGE ( 'NONE', *, *, #18995, .T. ) ;
#10490=DIRECTION ( 'NONE',  ( 1.000000000000000000, 4.708535149079844747E-14, 3.717264591378824873E-16 ) ) ;
#10491=DIRECTION ( 'NONE',  ( 3.330669073875432643E-16, 4.437342591868153746E-31, -1.000000000000000000 ) ) ;
#10492=DIRECTION ( 'NONE',  ( -1.000000000000000000, -2.699383410053119644E-30, -3.330669073875432643E-16 ) ) ;
#10497=DIRECTION ( 'NONE',  ( -3.885780586188016830E-16, -4.437342591868156373E-31, 1.000000000000000000 ) ) ;
#10498=CARTESIAN_POINT ( 'NONE',  ( 119.5756419024615838, -11.00000000000006573, -6.000000000000116351 ) ) ;
#10507=DIRECTION ( 'NONE',  ( -1.000000000000000000, -2.699383410053118943E-30, -2.668805347656595124E-16 ) ) ;
#10508=LINE ( 'NONE', #3232, #8525 ) ;
#10515=ORIENTED_EDGE ( 'NONE', *, *, #12242, .F. ) ;
#10522=ADVANCED_FACE ( 'NONE', ( #5422 ), #15, .T. ) ;
#10540=CARTESIAN_POINT ( 'NONE',  ( 116.8476484622116232, -8.074585193523331483, 6.500000000000040856 ) ) ;
#10542=ORIENTED_EDGE ( 'NONE', *, *, #11284, .F. ) ;
#10547=DIRECTION ( 'NONE',  ( -1.000000000000000000, 0.000000000000000000, -4.336808689941968432E-16 ) ) ;
#10549=EDGE_CURVE ( 'NONE', #20921, #21696, #18921, .T. ) ;
#10561=DIRECTION ( 'NONE',  ( 0.7313537016191735685, -0.6819983600624951459, 3.923113172947598083E-16 ) ) ;
#10563=DIRECTION ( 'NONE',  ( 0.7313537016191746787, 0.6819983600624940356, 1.072890437865584409E-16 ) ) ;
#10566=VERTEX_POINT ( 'NONE', #7521 ) ;
#10574=DIRECTION ( 'NONE',  ( 3.032184104443272185E-30, 1.000000000000000000, -7.395570986447005381E-32 ) ) ;
#10575=EDGE_CURVE ( 'NONE', #11319, #18271, #17796, .T. ) ;
#10599=ADVANCED_FACE ( 'NONE', ( #3862 ), #18167, .T. ) ;
#10611=DIRECTION ( 'NONE',  ( 0.7313537016191730133, -0.6819983600624958120, 5.924440990721418971E-17 ) ) ;
#10616=EDGE_CURVE ( 'NONE', #1495, #15578, #701, .T. ) ;
#10635=CARTESIAN_POINT ( 'NONE',  ( 63.50658097017375070, -4.500000000000003553, 6.000000000000185629 ) ) ;
#10647=VECTOR ( 'NONE', #5766, 1000.000000000000000 ) ;
#10655=ADVANCED_FACE ( 'NONE', ( #354 ), #11384, .F. ) ;
#10663=ORIENTED_EDGE ( 'NONE', *, *, #15451, .T. ) ;
#10679=DIRECTION ( 'NONE',  ( 0.000000000000000000, 1.000000000000000000, 0.000000000000000000 ) ) ;
#10685=AXIS2_PLACEMENT_3D ( 'NONE', #21772, #589, #9293 ) ;
#10687=ORIENTED_EDGE ( 'NONE', *, *, #1522, .T. ) ;
#10693=DIRECTION ( 'NONE',  ( 3.885780586188016830E-16, 4.437342591868156373E-31, -1.000000000000000000 ) ) ;
#10707=EDGE_CURVE ( 'NONE', #23176, #9421, #6576, .T. ) ;
#10710=ORIENTED_EDGE ( 'NONE', *, *, #1892, .T. ) ;
#10711=AXIS2_PLACEMENT_3D ( 'NONE', #4325, #2572, #7988 ) ;
#10718=ORIENTED_EDGE ( 'NONE', *, *, #2593, .F. ) ;
#10734=EDGE_CURVE ( 'NONE', #13735, #13332, #10201, .T. ) ;
#10749=ORIENTED_EDGE ( 'NONE', *, *, #3887, .F. ) ;
#10767=TOROIDAL_SURFACE ( 'NONE', #11511, 4.500000000000000888, 0.5000000000000000000 ) ;
#10768=CARTESIAN_POINT ( 'NONE',  ( 88.75737332930594903, -6.527605602963476805, 6.500000000000151879 ) ) ;
#10786=CARTESIAN_POINT ( 'NONE',  ( 66.26395429947839943, 0.000000000000000000, 6.000000000000178524 ) ) ;
#10790=MECHANICAL_DESIGN_GEOMETRIC_PRESENTATION_REPRESENTATION('',(#5908),#16400);
#10802=EDGE_CURVE ( 'NONE', #17658, #14732, #13296, .T. ) ;
#10810=EDGE_CURVE ( 'NONE', #8517, #15515, #2921, .T. ) ;
#10811=DIRECTION ( 'NONE',  ( -1.000000000000000000, 0.000000000000000000, -3.717264591378832268E-16 ) ) ;
#10814=DIRECTION ( 'NONE',  ( -0.6819983600624998088, -0.7313537016191693496, 0.000000000000000000 ) ) ;
#10826=ORIENTED_EDGE ( 'NONE', *, *, #8855, .F. ) ;
#10860=ORIENTED_EDGE ( 'NONE', *, *, #12556, .F. ) ;
#10869=EDGE_CURVE ( 'NONE', #5312, #20860, #1617, .T. ) ;
#10875=DIRECTION ( 'NONE',  ( 0.7313537016191730133, -0.6819983600624959230, 5.924440990721418971E-17 ) ) ;
#10879=ORIENTED_EDGE ( 'NONE', *, *, #979, .F. ) ;
#10885=ORIENTED_EDGE ( 'NONE', *, *, #9307, .T. ) ;
#10900=DIRECTION ( 'NONE',  ( 3.885780586188016830E-16, 4.437342591868156373E-31, -1.000000000000000000 ) ) ;
#10907=CARTESIAN_POINT ( 'NONE',  ( 61.83096495907203405, -4.753799060524588782, -5.999999999999956479 ) ) ;
#10912=LINE ( 'NONE', #7298, #21989 ) ;
#10913=VERTEX_POINT ( 'NONE', #8912 ) ;
#10917=CYLINDRICAL_SURFACE ( 'NONE', #18188, 0.4999999999999978351 ) ;
#10930=EDGE_CURVE ( 'NONE', #9421, #13451, #2717, .T. ) ;
#10932=ORIENTED_EDGE ( 'NONE', *, *, #8072, .F. ) ;
#10934=EDGE_LOOP ( 'NONE', ( #15216, #3184, #2721, #13591 ) ) ;
#10939=DIRECTION ( 'NONE',  ( -3.032184104443272185E-30, -1.000000000000000000, 7.395570986447005381E-32 ) ) ;
#10946=EDGE_CURVE ( 'NONE', #15916, #21787, #9868, .T. ) ;
#10952=CARTESIAN_POINT ( 'NONE',  ( 66.26395429947831417, -4.500000000000003553, 6.000000000000192735 ) ) ;
#10953=FACE_BOUND ( 'NONE', #16951, .T. ) ;
#10969=ORIENTED_EDGE ( 'NONE', *, *, #6232, .F. ) ;
#10984=CARTESIAN_POINT ( 'NONE',  ( 108.2426266706970637, -13.52760560296348302, 6.500000000000019540 ) ) ;
#10987=DIRECTION ( 'NONE',  ( -1.000000000000000000, -2.699383410053119644E-30, -3.330669073875432643E-16 ) ) ;
#11000=AXIS2_PLACEMENT_3D ( 'NONE', #1436, #20865, #11899 ) ;
#11005=DIRECTION ( 'NONE',  ( -3.330669073875432643E-16, -4.437342591868153746E-31, 1.000000000000000000 ) ) ;
#11021=LINE ( 'NONE', #14668, #3287 ) ;
#11026=ORIENTED_EDGE ( 'NONE', *, *, #5139, .T. ) ;
#11028=AXIS2_PLACEMENT_3D ( 'NONE', #795, #20440, #6204 ) ;
#11060=ORIENTED_EDGE ( 'NONE', *, *, #788, .F. ) ;
#11061=EDGE_LOOP ( 'NONE', ( #6753, #17778, #22968, #18973 ) ) ;
#11062=AXIS2_PLACEMENT_3D ( 'NONE', #2621, #9797, #4732 ) ;
#11078=LINE ( 'NONE', #14502, #15679 ) ;
#11079=EDGE_CURVE ( 'NONE', #9470, #10566, #210, .T. ) ;
#11089=EDGE_LOOP ( 'NONE', ( #20942, #6784 ) ) ;
#11092=EDGE_CURVE ( 'NONE', #10216, #16775, #6110, .T. ) ;
#11104=LINE ( 'NONE', #79, #7390 ) ;
#11110=DIRECTION ( 'NONE',  ( 0.000000000000000000, 0.000000000000000000, 1.000000000000000000 ) ) ;
#11127=EDGE_CURVE ( 'NONE', #17658, #6130, #3844, .T. ) ;
#11136=CIRCLE ( 'NONE', #15271, 0.4999999999999990563 ) ;
#11142=( NAMED_UNIT ( * ) SI_UNIT ( $, .STERADIAN. ) SOLID_ANGLE_UNIT ( ) );
#11145=CIRCLE ( 'NONE', #1758, 0.5000000000000038858 ) ;
#11157=VECTOR ( 'NONE', #8746, 1000.000000000000000 ) ;
#11159=DIRECTION ( 'NONE',  ( 3.885780586188016830E-16, 4.437342591868156373E-31, -1.000000000000000000 ) ) ;
#11174=ORIENTED_EDGE ( 'NONE', *, *, #20779, .F. ) ;
#11190=DIRECTION ( 'NONE',  ( 0.000000000000000000, 0.000000000000000000, 1.000000000000000000 ) ) ;
#11195=FILL_AREA_STYLE ('',( #2256 ) ) ;
#11197=CIRCLE ( 'NONE', #18341, 6.000000000000047962 ) ;
#11220=VECTOR ( 'NONE', #4621, 1000.000000000000000 ) ;
#11225=CARTESIAN_POINT ( 'NONE',  ( 77.42435809754140053, -10.99999999999981526, -6.499999999999999112 ) ) ;
#11226=LINE ( 'NONE', #9351, #3889 ) ;
#11236=ORIENTED_EDGE ( 'NONE', *, *, #10802, .F. ) ;
#11240=ORIENTED_EDGE ( 'NONE', *, *, #8114, .T. ) ;
#11246=AXIS2_PLACEMENT_3D ( 'NONE', #22979, #3335, #17667 ) ;
#11253=CARTESIAN_POINT ( 'NONE',  ( 63.53596085922836068, -2.925414806476678287, 6.500000000000123457 ) ) ;
#11255=AXIS2_PLACEMENT_3D ( 'NONE', #17104, #11159, #13165 ) ;
#11257=DIRECTION ( 'NONE',  ( 1.000000000000000000, -1.847414967615758933E-47, 3.885780586188017323E-16 ) ) ;
#11262=ADVANCED_FACE ( 'NONE', ( #17466 ), #1474, .T. ) ;
#11263=ORIENTED_EDGE ( 'NONE', *, *, #10616, .T. ) ;
#11265=DIRECTION ( 'NONE',  ( -0.6819983600625064701, -0.7313537016191632434, 0.000000000000000000 ) ) ;
#11273=CARTESIAN_POINT ( 'NONE',  ( 54.42435809754113052, -4.000000000000003553, -6.499999999999999112 ) ) ;
#11275=PLANE ( 'NONE',  #6441 ) ;
#11278=CARTESIAN_POINT ( 'NONE',  ( 63.19496167919701435, -3.291091657286332683, -6.499999999999970690 ) ) ;
#11280=CARTESIAN_POINT ( 'NONE',  ( 124.5000000000019469, -13.52760560296373171, -6.938893903907228378E-15 ) ) ;
#11284=EDGE_CURVE ( 'NONE', #15739, #12056, #20399, .T. ) ;
#11298=CARTESIAN_POINT ( 'NONE',  ( 86.02937988905577527, -9.453020409440155092, -5.999999999999991118 ) ) ;
#11299=CARTESIAN_POINT ( 'NONE',  ( 77.42435809754137210, -6.999999999999811706, 6.000000000000088818 ) ) ;
#11302=PRESENTATION_STYLE_ASSIGNMENT (( #9779 ) ) ;
#11319=VERTEX_POINT ( 'NONE', #23252 ) ;
#11324=EDGE_CURVE ( 'NONE', #8293, #6969, #17695, .T. ) ;
#11326=DIRECTION ( 'NONE',  ( 0.6819983600624981435, -0.7313537016191709039, 0.000000000000000000 ) ) ;
#11332=CARTESIAN_POINT ( 'NONE',  ( 82.19834661797897013, -5.880524088665628923, 6.000000000000109246 ) ) ;
#11340=CIRCLE ( 'NONE', #23000, 6.500000000000061284 ) ;
#11343=VERTEX_POINT ( 'NONE', #8535 ) ;
#11347=DIRECTION ( 'NONE',  ( -3.885780586188016830E-16, -4.437342591868156373E-31, 1.000000000000000000 ) ) ;
#11374=EDGE_LOOP ( 'NONE', ( #12773, #22759, #1128, #12412 ) ) ;
#11375=AXIS2_PLACEMENT_3D ( 'NONE', #7437, #14606, #20133 ) ;
#11384=CYLINDRICAL_SURFACE ( 'NONE', #16646, 2.550000000000012701 ) ;
#11398=AXIS2_PLACEMENT_3D ( 'NONE', #2331, #2451, #21990 ) ;
#11400=VECTOR ( 'NONE', #3530, 1000.000000000000000 ) ;
#11403=EDGE_CURVE ( 'NONE', #18644, #7880, #291, .T. ) ;
#11409=CIRCLE ( 'NONE', #11028, 0.5000000000000038858 ) ;
#11421=CARTESIAN_POINT ( 'NONE',  ( 6.500000000000339284, 0.5000000000001947331, 6.500000000000130562 ) ) ;
#11423=( LENGTH_UNIT ( ) NAMED_UNIT ( * ) SI_UNIT ( .MILLI., .METRE. ) );
#11432=VERTEX_POINT ( 'NONE', #9461 ) ;
#11435=VERTEX_POINT ( 'NONE', #12874 ) ;
#11440=CARTESIAN_POINT ( 'NONE',  ( 54.42435809754113052, -4.000000000000003553, -6.000000000000012434 ) ) ;
#11443=DIRECTION ( 'NONE',  ( 0.000000000000000000, 0.000000000000000000, 1.000000000000000000 ) ) ;
#11450=CARTESIAN_POINT ( 'NONE',  ( 59.19834661797874986, 1.119475911334072427, -5.999999999999908518 ) ) ;
#11453=PLANE ( 'NONE',  #7790 ) ;
#11460=ORIENTED_EDGE ( 'NONE', *, *, #12932, .T. ) ;
#11466=DIRECTION ( 'NONE',  ( -0.7313537016191767881, -0.6819983600624918152, -4.403559511741033569E-16 ) ) ;
#11469=DIRECTION ( 'NONE',  ( 0.000000000000000000, -1.000000000000000000, 0.000000000000000000 ) ) ;
#11482=EDGE_LOOP ( 'NONE', ( #23002, #801, #21391, #22876 ) ) ;
#11485=ORIENTED_EDGE ( 'NONE', *, *, #20917, .T. ) ;
#11492=VECTOR ( 'NONE', #21628, 1000.000000000000114 ) ;
#11502=TOROIDAL_SURFACE ( 'NONE', #7031, 4.500000000000000888, 0.5000000000000000000 ) ;
#11511=AXIS2_PLACEMENT_3D ( 'NONE', #11440, #18507, #2734 ) ;
#11516=VERTEX_POINT ( 'NONE', #20403 ) ;
#11530=CARTESIAN_POINT ( 'NONE',  ( 54.42435809754118736, 0.4999999999999449329, -6.499999999999922728 ) ) ;
#11531=CARTESIAN_POINT ( 'NONE',  ( 77.42435809754135789, -10.99999999999981526, 6.500000000000123457 ) ) ;
#11543=VERTEX_POINT ( 'NONE', #15082 ) ;
#11552=ORIENTED_EDGE ( 'NONE', *, *, #18193, .F. ) ;
#11564=AXIS2_PLACEMENT_3D ( 'NONE', #6487, #13668, #20855 ) ;
#11573=ORIENTED_EDGE ( 'NONE', *, *, #22746, .F. ) ;
#11582=EDGE_CURVE ( 'NONE', #3321, #23117, #20418, .T. ) ;
#11599=ORIENTED_EDGE ( 'NONE', *, *, #15551, .T. ) ;
#11602=CARTESIAN_POINT ( 'NONE',  ( 55.36587326203805048, 4.009651402420072230, -5.999999999999963585 ) ) ;
#11609=TOROIDAL_SURFACE ( 'NONE', #21415, 4.500000000000000888, 0.5000000000000000000 ) ;
#11614=CARTESIAN_POINT ( 'NONE',  ( 108.9540049198142100, -11.33354449810611264, 6.000000000000088818 ) ) ;
#11615=DIRECTION ( 'NONE',  ( -1.000000000000000000, 1.847414967615758933E-47, -3.885780586188017323E-16 ) ) ;
#11618=VECTOR ( 'NONE', #15518, 1000.000000000000114 ) ;
#11626=DIRECTION ( 'NONE',  ( -5.598259082250079541E-17, 1.000000000000000000, -6.162975822039171151E-32 ) ) ;
#11628=CARTESIAN_POINT ( 'NONE',  ( 77.42435809754140053, -6.999999999999811706, -5.999999999999984901 ) ) ;
#11632=ORIENTED_EDGE ( 'NONE', *, *, #16277, .F. ) ;
#11641=DIRECTION ( 'NONE',  ( 3.885780586188016830E-16, 4.437342591868156373E-31, -1.000000000000000000 ) ) ;
#11645=DIRECTION ( 'NONE',  ( 0.6819983600624998088, 0.7313537016191693496, 0.000000000000000000 ) ) ;
#11657=ORIENTED_EDGE ( 'NONE', *, *, #10549, .T. ) ;
#11680=CARTESIAN_POINT ( 'NONE',  ( 108.2426266706970779, -6.527605602963587828, 6.000000000000109246 ) ) ;
#11683=CARTESIAN_POINT ( 'NONE',  ( 80.15235153779138955, -8.074585193523137860, 6.500000000000040856 ) ) ;
#11688=ORIENTED_EDGE ( 'NONE', *, *, #18000, .F. ) ;
#11689=VERTEX_POINT ( 'NONE', #19683 ) ;
#11702=CARTESIAN_POINT ( 'NONE',  ( 6.500000000000283329, 1.942890293094023946E-13, -5.999999999999943157 ) ) ;
#11711=CARTESIAN_POINT ( 'NONE',  ( 109.3164911904586774, -11.67918431276168612, -6.500000000000054179 ) ) ;
#11712=ORIENTED_EDGE ( 'NONE', *, *, #9301, .T. ) ;
#11732=DIRECTION ( 'NONE',  ( 3.885780586188016830E-16, 4.437342591868156373E-31, -1.000000000000000000 ) ) ;
#11756=ORIENTED_EDGE ( 'NONE', *, *, #3043, .F. ) ;
#11757=CARTESIAN_POINT ( 'NONE',  ( 124.5000000000018332, -4.000000000000058620, -5.999999999999943157 ) ) ;
#11760=ORIENTED_EDGE ( 'NONE', *, *, #10869, .T. ) ;
#11767=CYLINDRICAL_SURFACE ( 'NONE', #821, 0.4999999999999978351 ) ;
#11768=TOROIDAL_SURFACE ( 'NONE', #1634, 4.500000000000000888, 0.5000000000000000000 ) ;
#11769=DIRECTION ( 'NONE',  ( -0.6819983600624981435, -0.7313537016191709039, 0.000000000000000000 ) ) ;
#11774=VECTOR ( 'NONE', #5524, 1000.000000000000000 ) ;
#11782=EDGE_CURVE ( 'NONE', #4634, #8517, #2129, .T. ) ;
#11785=ORIENTED_EDGE ( 'NONE', *, *, #14191, .F. ) ;
#11788=DIRECTION ( 'NONE',  ( 3.885780586188016830E-16, 4.437342591868156373E-31, -1.000000000000000000 ) ) ;
#11791=LINE ( 'NONE', #18978, #1311 ) ;
#11800=CARTESIAN_POINT ( 'NONE',  ( 63.19496167919710672, -3.291091657286276728, 6.000000000000123457 ) ) ;
#11807=CARTESIAN_POINT ( 'NONE',  ( 88.75737332930592061, -6.527605602963476805, -6.000000000000012434 ) ) ;
#11808=DIRECTION ( 'NONE',  ( 1.000000000000000000, 1.421085471520213625E-14, 3.854941057726199147E-16 ) ) ;
#11813=ORIENTED_EDGE ( 'NONE', *, *, #1210, .F. ) ;
#11830=CARTESIAN_POINT ( 'NONE',  ( 108.2426266706970637, -13.02760560296359316, 5.999999999999984901 ) ) ;
#11839=EDGE_CURVE ( 'NONE', #10566, #16898, #19276, .T. ) ;
#11841=VECTOR ( 'NONE', #14571, 1000.000000000000000 ) ;
#11853=CARTESIAN_POINT ( 'NONE',  ( 77.42435809754140053, -6.999999999999811706, -5.999999999999984901 ) ) ;
#11879=LINE ( 'NONE', #13993, #18769 ) ;
#11892=VECTOR ( 'NONE', #22429, 1000.000000000000000 ) ;
#11898=ORIENTED_EDGE ( 'NONE', *, *, #7242, .F. ) ;
#11899=DIRECTION ( 'NONE',  ( -0.6819983600625061371, -0.7313537016191633544, 0.000000000000000000 ) ) ;
#11902=CARTESIAN_POINT ( 'NONE',  ( 66.26395429947839943, 0.000000000000000000, 6.000000000000178524 ) ) ;
#11921=EDGE_LOOP ( 'NONE', ( #18795, #11263, #1157, #2552 ) ) ;
#11931=DIRECTION ( 'NONE',  ( 3.330669073875432643E-16, 4.437342591868153746E-31, -1.000000000000000000 ) ) ;
#11937=CARTESIAN_POINT ( 'NONE',  ( 57.15235153779114796, -1.074585193523325266, -6.499999999999977796 ) ) ;
#11948=AXIS2_PLACEMENT_3D ( 'NONE', #15297, #1421, #8596 ) ;
#11954=ORIENTED_EDGE ( 'NONE', *, *, #8532, .T. ) ;
#11980=CIRCLE ( 'NONE', #14990, 4.500000000000045297 ) ;
#11984=ORIENTED_EDGE ( 'NONE', *, *, #20586, .F. ) ;
#12004=EDGE_LOOP ( 'NONE', ( #13168, #14883, #22233, #6907 ) ) ;
#12013=DIRECTION ( 'NONE',  ( -1.000000000000000000, -2.699383410053117892E-30, -3.885780586188017323E-16 ) ) ;
#12024=CARTESIAN_POINT ( 'NONE',  ( 6.500000000000283329, 3.000000000000141220, -5.999999999999943157 ) ) ;
#12034=EDGE_LOOP ( 'NONE', ( #22177, #4493, #19546, #10718 ) ) ;
#12044=DIRECTION ( 'NONE',  ( 0.6819983600625073583, -0.7313537016191622442, -1.665472943098395307E-16 ) ) ;
#12047=DIRECTION ( 'NONE',  ( -1.000000000000000000, -2.699383410053119644E-30, -3.330669073875432643E-16 ) ) ;
#12056=VERTEX_POINT ( 'NONE', #4313 ) ;
#12071=ADVANCED_FACE ( 'NONE', ( #6217 ), #18940, .T. ) ;
#12075=TOROIDAL_SURFACE ( 'NONE', #16587, 4.500000000000000888, 0.5000000000000000000 ) ;
#12081=EDGE_CURVE ( 'NONE', #6130, #18644, #5411, .T. ) ;
#12089=VERTEX_POINT ( 'NONE', #6571 ) ;
#12094=PLANE ( 'NONE',  #3225 ) ;
#12097=ADVANCED_FACE ( 'NONE', ( #13738 ), #10196, .T. ) ;
#12100=DIRECTION ( 'NONE',  ( 0.000000000000000000, 0.000000000000000000, 1.000000000000000000 ) ) ;
#12117=EDGE_CURVE ( 'NONE', #13355, #16151, #4257, .T. ) ;
#12127=ORIENTED_EDGE ( 'NONE', *, *, #13063, .T. ) ;
#12147=CARTESIAN_POINT ( 'NONE',  ( 61.48996577904083694, -5.119475911334187224, 6.500000000000130562 ) ) ;
#12149=CIRCLE ( 'NONE', #23078, 0.5000000000000038858 ) ;
#12155=AXIS2_PLACEMENT_3D ( 'NONE', #20077, #3828, #22069 ) ;
#12161=CARTESIAN_POINT ( 'NONE',  ( 114.8016533820240852, -5.880524088665822546, 6.000000000000123457 ) ) ;
#12163=DIRECTION ( 'NONE',  ( -1.000000000000000000, -2.699383410053119644E-30, -3.330669073875432643E-16 ) ) ;
#12170=CARTESIAN_POINT ( 'NONE',  ( 119.5756419024615553, -11.00000000000006573, 6.500000000000012434 ) ) ;
#12172=AXIS2_PLACEMENT_3D ( 'NONE', #4287, #11466, #2531 ) ;
#12173=CARTESIAN_POINT ( 'NONE',  ( 118.0000000000018190, -4.500000000000003553, 6.000000000000109246 ) ) ;
#12176=DIRECTION ( 'NONE',  ( -1.000000000000000000, -5.598259082250514647E-17, -3.330669073875432643E-16 ) ) ;
#12179=CARTESIAN_POINT ( 'NONE',  ( 88.75737332930587797, -11.02760560296348125, -6.000000000000067502 ) ) ;
#12187=DIRECTION ( 'NONE',  ( -3.885780586188016830E-16, -4.437342591868156373E-31, 1.000000000000000000 ) ) ;
#12190=DIRECTION ( 'NONE',  ( 1.000000000000000000, 0.000000000000000000, 2.668805347656601040E-16 ) ) ;
#12201=EDGE_CURVE ( 'NONE', #18645, #16059, #8908, .T. ) ;
#12204=ORIENTED_EDGE ( 'NONE', *, *, #10810, .T. ) ;
#12205=ORIENTED_EDGE ( 'NONE', *, *, #766, .T. ) ;
#12208=VERTEX_POINT ( 'NONE', #19607 ) ;
#12224=ADVANCED_FACE ( 'NONE', ( #5018 ), #21034, .F. ) ;
#12235=EDGE_LOOP ( 'NONE', ( #3113, #4573, #22825, #10879 ) ) ;
#12242=EDGE_CURVE ( 'NONE', #12089, #8376, #15531, .T. ) ;
#12243=CARTESIAN_POINT ( 'NONE',  ( 118.0000000000017195, -4.000000000000003553, 6.500000000000130562 ) ) ;
#12258=ORIENTED_EDGE ( 'NONE', *, *, #12117, .T. ) ;
#12259=ADVANCED_FACE ( 'NONE', ( #19957 ), #21960, .T. ) ;
#12263=EDGE_CURVE ( 'NONE', #3634, #9737, #22315, .T. ) ;
#12270=ORIENTED_EDGE ( 'NONE', *, *, #23074, .T. ) ;
#12271=CARTESIAN_POINT ( 'NONE',  ( 108.2426266706972058, -6.527605602963671316, -6.500000000000019540 ) ) ;
#12275=VERTEX_POINT ( 'NONE', #19842 ) ;
#12284=LINE ( 'NONE', #17347, #19586 ) ;
#12286=DIRECTION ( 'NONE',  ( -1.000000000000000000, -2.699383410053119644E-30, -3.330669073875432643E-16 ) ) ;
#12293=FACE_OUTER_BOUND ( 'NONE', #15510, .T. ) ;
#12297=CIRCLE ( 'NONE', #5932, 0.5000000000000038858 ) ;
#12331=AXIS2_PLACEMENT_3D ( 'NONE', #7929, #20408, #6408 ) ;
#12332=CIRCLE ( 'NONE', #23265, 2.550000000000024691 ) ;
#12353=EDGE_LOOP ( 'NONE', ( #11240, #21141, #3767, #21958 ) ) ;
#12361=EDGE_LOOP ( 'NONE', ( #284, #5614, #13470, #21474 ) ) ;
#12373=ADVANCED_FACE ( 'NONE', ( #1946 ), #14433, .T. ) ;
#12378=ADVANCED_FACE ( 'NONE', ( #7601 ), #16305, .T. ) ;
#12380=DIRECTION ( 'NONE',  ( 1.000000000000000000, 4.972873964466789154E-14, 3.854941057726193231E-16 ) ) ;
#12386=ORIENTED_EDGE ( 'NONE', *, *, #8990, .T. ) ;
#12396=ORIENTED_EDGE ( 'NONE', *, *, #6362, .F. ) ;
#12397=DIRECTION ( 'NONE',  ( -1.000000000000000000, 0.000000000000000000, -2.668805347656595124E-16 ) ) ;
#12406=DIRECTION ( 'NONE',  ( -1.000000000000000000, -2.699383410053119644E-30, -3.330669073875432643E-16 ) ) ;
#12409=DIRECTION ( 'NONE',  ( 0.000000000000000000, 0.000000000000000000, 1.000000000000000000 ) ) ;
#12412=ORIENTED_EDGE ( 'NONE', *, *, #1086, .T. ) ;
#12415=CARTESIAN_POINT ( 'NONE',  ( 88.75737332930596324, -6.527605602963476805, 6.000000000000165201 ) ) ;
#12424=DIRECTION ( 'NONE',  ( 3.032184104443272185E-30, 1.000000000000000000, -7.395570986447005381E-32 ) ) ;
#12474=ORIENTED_EDGE ( 'NONE', *, *, #9226, .T. ) ;
#12500=ORIENTED_EDGE ( 'NONE', *, *, #5927, .F. ) ;
#12502=CIRCLE ( 'NONE', #22664, 0.5000000000000018874 ) ;
#12510=CIRCLE ( 'NONE', #3855, 0.4999999999999984457 ) ;
#12519=CARTESIAN_POINT ( 'NONE',  ( 66.26395429947832838, -7.000000000000006217, 6.000000000000172307 ) ) ;
#12524=VECTOR ( 'NONE', #22108, 1000.000000000000000 ) ;
#12529=AXIS2_PLACEMENT_3D ( 'NONE', #21182, #17876, #19284 ) ;
#12537=EDGE_CURVE ( 'NONE', #8293, #16898, #20451, .T. ) ;
#12543=TOROIDAL_SURFACE ( 'NONE', #14044, 4.500000000000000888, 0.5000000000000000000 ) ;
#12549=DIRECTION ( 'NONE',  ( 0.6819983600625055820, 0.7313537016191637985, 4.996142016973858765E-16 ) ) ;
#12555=LINE ( 'NONE', #21406, #12968 ) ;
#12556=EDGE_CURVE ( 'NONE', #14050, #19728, #18953, .T. ) ;
#12561=PLANE ( 'NONE',  #22117 ) ;
#12563=AXIS2_PLACEMENT_3D ( 'NONE', #6257, #6602, #13776 ) ;
#12578=ORIENTED_EDGE ( 'NONE', *, *, #11079, .F. ) ;
#12580=DIRECTION ( 'NONE',  ( 3.885780586188016830E-16, 4.437342591868156373E-31, -1.000000000000000000 ) ) ;
#12588=DIRECTION ( 'NONE',  ( 3.885780586188016830E-16, 4.437342591868156373E-31, -1.000000000000000000 ) ) ;
#12598=EDGE_LOOP ( 'NONE', ( #8554, #5828, #17991, #1668 ) ) ;
#12599=EDGE_LOOP ( 'NONE', ( #4395, #22816, #19489, #21085 ) ) ;
#12607=CARTESIAN_POINT ( 'NONE',  ( 108.2426266706971205, -13.02760560296367665, -6.500000000000075495 ) ) ;
#12612=AXIS2_PLACEMENT_3D ( 'NONE', #5321, #21565, #12722 ) ;
#12621=UNCERTAINTY_MEASURE_WITH_UNIT (LENGTH_MEASURE( 1.000000000000000082E-05 ), #22203, 'distance_accuracy_value', 'NONE');
#12627=ORIENTED_EDGE ( 'NONE', *, *, #9230, .F. ) ;
#12630=VECTOR ( 'NONE', #10693, 1000.000000000000000 ) ;
#12631=CARTESIAN_POINT ( 'NONE',  ( 119.5756419024615838, -6.500000000000061284, -6.499999999999992006 ) ) ;
#12652=VECTOR ( 'NONE', #7333, 1000.000000000000000 ) ;
#12666=CARTESIAN_POINT ( 'NONE',  ( 85.68838070902457105, -9.818697260249752645, -6.500000000000019540 ) ) ;
#12668=ADVANCED_FACE ( 'NONE', ( #5111 ), #22766, .T. ) ;
#12678=ORIENTED_EDGE ( 'NONE', *, *, #13859, .F. ) ;
#12689=CARTESIAN_POINT ( 'NONE',  ( 88.75737332930587797, -10.52760560296347947, 6.500000000000075495 ) ) ;
#12709=CARTESIAN_POINT ( 'NONE',  ( 54.42435809754115894, 2.499999999999946709, -5.999999999999950262 ) ) ;
#12715=ORIENTED_EDGE ( 'NONE', *, *, #11127, .T. ) ;
#12716=EDGE_CURVE ( 'NONE', #6413, #12275, #7696, .T. ) ;
#12718=ORIENTED_EDGE ( 'NONE', *, *, #18193, .T. ) ;
#12722=DIRECTION ( 'NONE',  ( -1.000000000000000000, 1.511687600494058571E-14, -3.717264591378832268E-16 ) ) ;
#12726=DIRECTION ( 'NONE',  ( 3.885780586188016830E-16, 4.437342591868156373E-31, -1.000000000000000000 ) ) ;
#12733=DIRECTION ( 'NONE',  ( -3.885780586188016830E-16, -4.437342591868156373E-31, 1.000000000000000000 ) ) ;
#12746=EDGE_LOOP ( 'NONE', ( #14202, #13033, #417, #13182 ) ) ;
#12753=CARTESIAN_POINT ( 'NONE',  ( 88.75737332930597745, -13.02760560296348302, 6.500000000000103029 ) ) ;
#12763=CARTESIAN_POINT ( 'NONE',  ( 124.5000000000018332, -4.500000000000087041, -6.499999999999964473 ) ) ;
#12773=ORIENTED_EDGE ( 'NONE', *, *, #2040, .T. ) ;
#12781=VECTOR ( 'NONE', #18252, 1000.000000000000000 ) ;
#12783=LINE ( 'NONE', #324, #593 ) ;
#12799=EDGE_LOOP ( 'NONE', ( #3603, #12270, #21388, #1573 ) ) ;
#12800=ADVANCED_FACE ( 'NONE', ( #13099 ), #17936, .T. ) ;
#12802=DIRECTION ( 'NONE',  ( 3.885780586188016830E-16, 4.437342591868156373E-31, -1.000000000000000000 ) ) ;
#12809=CARTESIAN_POINT ( 'NONE',  ( 73.50000000000112266, -3.999999999999809042, 1.179611963664228824E-13 ) ) ;
#12811=CARTESIAN_POINT ( 'NONE',  ( 108.2426266706970637, -13.02760560296348302, 6.500000000000019540 ) ) ;
#12816=CARTESIAN_POINT ( 'NONE',  ( 77.42435809754145737, -3.999999999999809042, -6.499999999999984901 ) ) ;
#12829=VECTOR ( 'NONE', #1676, 1000.000000000000000 ) ;
#12830=ADVANCED_FACE ( 'NONE', ( #18504 ), #14973, .T. ) ;
#12831=DIRECTION ( 'NONE',  ( -3.330669073875432643E-16, -4.437342591868153746E-31, 1.000000000000000000 ) ) ;
#12833=CARTESIAN_POINT ( 'NONE',  ( 118.0000000000017479, -4.000000000000058620, -5.999999999999908518 ) ) ;
#12844=EDGE_CURVE ( 'NONE', #14050, #16775, #11791, .T. ) ;
#12847=ADVANCED_FACE ( 'NONE', ( #7918 ), #13564, .T. ) ;
#12848=LINE ( 'NONE', #7218, #4404 ) ;
#12850=CIRCLE ( 'NONE', #2332, 6.500000000000052403 ) ;
#12874=CARTESIAN_POINT ( 'NONE',  ( 59.19834661797869302, 1.119475911334100182, 6.000000000000165201 ) ) ;
#12878=AXIS2_PLACEMENT_3D ( 'NONE', #11531, #15643, #20611 ) ;
#12883=DIRECTION ( 'NONE',  ( 3.032184104443272185E-30, 1.000000000000000000, -7.395570986447005381E-32 ) ) ;
#12886=ORIENTED_EDGE ( 'NONE', *, *, #12888, .T. ) ;
#12888=EDGE_CURVE ( 'NONE', #522, #7130, #20747, .T. ) ;
#12889=VECTOR ( 'NONE', #12044, 1000.000000000000114 ) ;
#12895=ORIENTED_EDGE ( 'NONE', *, *, #4175, .T. ) ;
#12900=VECTOR ( 'NONE', #5155, 1000.000000000000000 ) ;
#12909=VECTOR ( 'NONE', #15886, 1000.000000000000000 ) ;
#12932=EDGE_CURVE ( 'NONE', #12208, #3270, #8396, .T. ) ;
#12937=AXIS2_PLACEMENT_3D ( 'NONE', #4716, #8595, #11769 ) ;
#12949=ORIENTED_EDGE ( 'NONE', *, *, #19168, .T. ) ;
#12950=TOROIDAL_SURFACE ( 'NONE', #2816, 4.500000000000000888, 0.5000000000000000000 ) ;
#12961=CYLINDRICAL_SURFACE ( 'NONE', #9581, 0.4999999999999978351 ) ;
#12967=CARTESIAN_POINT ( 'NONE',  ( 54.42435809754108078, -4.000000000000003553, 6.500000000000081712 ) ) ;
#12968=VECTOR ( 'NONE', #1511, 1000.000000000000114 ) ;
#12983=ORIENTED_EDGE ( 'NONE', *, *, #7095, .F. ) ;
#12988=EDGE_CURVE ( 'NONE', #21787, #12089, #6849, .T. ) ;
#12997=EDGE_CURVE ( 'NONE', #6421, #10139, #16650, .T. ) ;
#13001=ADVANCED_FACE ( 'NONE', ( #23100 ), #10372, .T. ) ;
#13006=CARTESIAN_POINT ( 'NONE',  ( 63.19496167919712093, -3.291091657286249195, 6.500000000000054179 ) ) ;
#13023=DIRECTION ( 'NONE',  ( -3.885780586188016830E-16, -4.437342591868156373E-31, 1.000000000000000000 ) ) ;
#13028=DIRECTION ( 'NONE',  ( -3.885780586188016830E-16, -4.437342591868156373E-31, 1.000000000000000000 ) ) ;
#13033=ORIENTED_EDGE ( 'NONE', *, *, #22180, .T. ) ;
#13058=VECTOR ( 'NONE', #5768, 1000.000000000000000 ) ;
#13063=EDGE_CURVE ( 'NONE', #8988, #4164, #18134, .T. ) ;
#13065=ORIENTED_EDGE ( 'NONE', *, *, #9354, .T. ) ;
#13076=CARTESIAN_POINT ( 'NONE',  ( 79.34099918003242635, -6.634323149190213265, -6.000000000000012434 ) ) ;
#13092=ORIENTED_EDGE ( 'NONE', *, *, #7052, .T. ) ;
#13099=FACE_OUTER_BOUND ( 'NONE', #18219, .T. ) ;
#13103=DIRECTION ( 'NONE',  ( 0.6819983600624989206, -0.7313537016191700157, 0.000000000000000000 ) ) ;
#13123=DIRECTION ( 'NONE',  ( -1.000000000000000000, 7.477632011778292156E-48, -3.885780586188017323E-16 ) ) ;
#13135=CARTESIAN_POINT ( 'NONE',  ( 73.50000000000116529, -3.999999999999809042, 2.550000000000110401 ) ) ;
#13140=DIRECTION ( 'NONE',  ( -3.885780586188016830E-16, -4.437342591868156373E-31, 1.000000000000000000 ) ) ;
#13145=VECTOR ( 'NONE', #22657, 1000.000000000000000 ) ;
#13161=LINE ( 'NONE', #12689, #11774 ) ;
#13164=CARTESIAN_POINT ( 'NONE',  ( 77.42435809754141474, -3.999999999999809042, 6.000000000000095923 ) ) ;
#13165=DIRECTION ( 'NONE',  ( -1.000000000000000000, 0.000000000000000000, -4.336808689941968432E-16 ) ) ;
#13168=ORIENTED_EDGE ( 'NONE', *, *, #12997, .T. ) ;
#13170=CARTESIAN_POINT ( 'NONE',  ( 119.5756419024616690, -7.000000000000062172, -6.500000000000033751 ) ) ;
#13182=ORIENTED_EDGE ( 'NONE', *, *, #6586, .T. ) ;
#13201=VECTOR ( 'NONE', #9381, 1000.000000000000000 ) ;
#13203=ORIENTED_EDGE ( 'NONE', *, *, #15817, .T. ) ;
#13208=ORIENTED_EDGE ( 'NONE', *, *, #2593, .T. ) ;
#13213=DIRECTION ( 'NONE',  ( -0.7313537016191755669, -0.6819983600624931475, 1.169467434532365146E-15 ) ) ;
#13225=DIRECTION ( 'NONE',  ( 3.885780586188016830E-16, 4.437342591868156373E-31, -1.000000000000000000 ) ) ;
#13243=FACE_OUTER_BOUND ( 'NONE', #14740, .T. ) ;
#13244=EDGE_CURVE ( 'NONE', #2907, #1495, #1303, .T. ) ;
#13264=ORIENTED_EDGE ( 'NONE', *, *, #20330, .F. ) ;
#13265=ORIENTED_EDGE ( 'NONE', *, *, #9860, .T. ) ;
#13268=CARTESIAN_POINT ( 'NONE',  ( 79.00000000000120792, -6.999999999999811706, 6.500000000000068390 ) ) ;
#13276=EDGE_CURVE ( 'NONE', #6044, #2907, #11879, .T. ) ;
#13278=AXIS2_PLACEMENT_3D ( 'NONE', #1332, #11788, #4844 ) ;
#13282=CARTESIAN_POINT ( 'NONE',  ( 84.32438398889952680, -11.28140466348806470, 6.500000000000137668 ) ) ;
#13296=CIRCLE ( 'NONE', #6919, 0.5000000000000038858 ) ;
#13304=FACE_OUTER_BOUND ( 'NONE', #11921, .T. ) ;
#13307=VERTEX_POINT ( 'NONE', #5058 ) ;
#13314=CYLINDRICAL_SURFACE ( 'NONE', #3823, 0.4999999999999978351 ) ;
#13323=EDGE_CURVE ( 'NONE', #15653, #16591, #17759, .T. ) ;
#13331=EDGE_LOOP ( 'NONE', ( #14728, #16259, #2145, #23147 ) ) ;
#13332=VERTEX_POINT ( 'NONE', #8940 ) ;
#13348=CARTESIAN_POINT ( 'NONE',  ( 119.5756419024615838, -11.00000000000006573, -6.500000000000075495 ) ) ;
#13355=VERTEX_POINT ( 'NONE', #16205 ) ;
#13366=FACE_OUTER_BOUND ( 'NONE', #17326, .T. ) ;
#13373=DIRECTION ( 'NONE',  ( -1.000000000000000000, -2.699383410053119644E-30, -3.330669073875432643E-16 ) ) ;
#13394=EDGE_CURVE ( 'NONE', #16867, #19367, #15380, .T. ) ;
#13402=DIRECTION ( 'NONE',  ( -0.7313537016191733464, 0.6819983600624954789, -3.733258675956564523E-18 ) ) ;
#13404=CARTESIAN_POINT ( 'NONE',  ( 124.5000000000019469, -7.000000000000062172, -2.549999999999971401 ) ) ;
#13422=DIRECTION ( 'NONE',  ( 1.000000000000000000, 2.699383410053119644E-30, 3.330669073875432643E-16 ) ) ;
#13432=DIRECTION ( 'NONE',  ( 3.032184104443272185E-30, 1.000000000000000000, -7.395570986447005381E-32 ) ) ;
#13433=AXIS2_PLACEMENT_3D ( 'NONE', #5161, #110, #7055 ) ;
#13435=VECTOR ( 'NONE', #7071, 1000.000000000000000 ) ;
#13438=VECTOR ( 'NONE', #21916, 1000.000000000000000 ) ;
#13443=EDGE_LOOP ( 'NONE', ( #19195, #3210, #15797, #5167 ) ) ;
#13447=EDGE_CURVE ( 'NONE', #7123, #17843, #22908, .T. ) ;
#13451=VERTEX_POINT ( 'NONE', #11702 ) ;
#13459=PLANE ( 'NONE',  #2538 ) ;
#13470=ORIENTED_EDGE ( 'NONE', *, *, #2235, .F. ) ;
#13475=AXIS2_PLACEMENT_3D ( 'NONE', #2231, #9414, #14815 ) ;
#13477=ORIENTED_EDGE ( 'NONE', *, *, #18050, .T. ) ;
#13478=EDGE_CURVE ( 'NONE', #11689, #10216, #8425, .T. ) ;
#13479=ORIENTED_EDGE ( 'NONE', *, *, #15983, .F. ) ;
#13485=DIRECTION ( 'NONE',  ( -3.885780586188016830E-16, -4.437342591868156373E-31, 1.000000000000000000 ) ) ;
#13486=DIRECTION ( 'NONE',  ( 1.000000000000000000, 1.776356839400265611E-14, 3.717264591378832268E-16 ) ) ;
#13513=VECTOR ( 'NONE', #21650, 1000.000000000000000 ) ;
#13514=DIRECTION ( 'NONE',  ( 3.032184104443272185E-30, 1.000000000000000000, -7.395570986447005381E-32 ) ) ;
#13526=ADVANCED_FACE ( 'NONE', ( #16670 ), #13599, .T. ) ;
#13527=CIRCLE ( 'NONE', #1145, 4.000000000000045297 ) ;
#13539=DIRECTION ( 'NONE',  ( -1.000000000000000000, -2.699383410053119644E-30, -3.330669073875432643E-16 ) ) ;
#13545=LINE ( 'NONE', #10233, #14395 ) ;
#13547=DIRECTION ( 'NONE',  ( -0.7313537016191752338, 0.6819983600624935915, -2.002134703001231171E-15 ) ) ;
#13564=PLANE ( 'NONE',  #6568 ) ;
#13575=DIRECTION ( 'NONE',  ( -1.000000000000000000, 0.000000000000000000, -2.668805347656595124E-16 ) ) ;
#13577=DIRECTION ( 'NONE',  ( -3.330669073875432643E-16, -4.437342591868153746E-31, 1.000000000000000000 ) ) ;
#13588=ORIENTED_EDGE ( 'NONE', *, *, #2829, .T. ) ;
#13591=ORIENTED_EDGE ( 'NONE', *, *, #13063, .F. ) ;
#13597=ORIENTED_EDGE ( 'NONE', *, *, #12988, .F. ) ;
#13599=PLANE ( 'NONE',  #19149 ) ;
#13604=DIRECTION ( 'NONE',  ( 1.000000000000000000, 0.000000000000000000, 2.668805347656595124E-16 ) ) ;
#13608=ADVANCED_FACE ( 'NONE', ( #21249 ), #4993, .T. ) ;
#13626=CARTESIAN_POINT ( 'NONE',  ( 80.15235153779146060, -8.074585193523137860, 6.000000000000109246 ) ) ;
#13630=CARTESIAN_POINT ( 'NONE',  ( 66.26395429947838522, 0.000000000000000000, 6.500000000000144773 ) ) ;
#13632=CIRCLE ( 'NONE', #3487, 4.500000000000045297 ) ;
#13651=DIRECTION ( 'NONE',  ( -3.330669073875432643E-16, -4.437342591868153746E-31, 1.000000000000000000 ) ) ;
#13653=ADVANCED_FACE ( 'NONE', ( #14176, #23130 ), #17940, .T. ) ;
#13655=ORIENTED_EDGE ( 'NONE', *, *, #8562, .T. ) ;
#13665=VECTOR ( 'NONE', #19733, 1000.000000000000114 ) ;
#13668=DIRECTION ( 'NONE',  ( 0.7313537016191731244, -0.6819983600624958120, 5.924440990721420203E-17 ) ) ;
#13672=ORIENTED_EDGE ( 'NONE', *, *, #1528, .F. ) ;
#13697=AXIS2_PLACEMENT_3D ( 'NONE', #13798, #15663, #22863 ) ;
#13705=ORIENTED_EDGE ( 'NONE', *, *, #18000, .T. ) ;
#13711=AXIS2_PLACEMENT_3D ( 'NONE', #21544, #3196, #10476 ) ;
#13713=EDGE_CURVE ( 'NONE', #7460, #11432, #13527, .T. ) ;
#13721=DIRECTION ( 'NONE',  ( -3.885780586188016830E-16, -4.437342591868156373E-31, 1.000000000000000000 ) ) ;
#13725=DIRECTION ( 'NONE',  ( 3.885780586188016830E-16, 4.437342591868156373E-31, -1.000000000000000000 ) ) ;
#13732=ORIENTED_EDGE ( 'NONE', *, *, #13478, .F. ) ;
#13733=EDGE_LOOP ( 'NONE', ( #7369, #1865 ) ) ;
#13735=VERTEX_POINT ( 'NONE', #287 ) ;
#13738=FACE_OUTER_BOUND ( 'NONE', #18825, .T. ) ;
#13745=ORIENTED_EDGE ( 'NONE', *, *, #13447, .F. ) ;
#13755=CARTESIAN_POINT ( 'NONE',  ( 61.48996577904083694, -5.119475911334187224, 6.000000000000067502 ) ) ;
#13756=VECTOR ( 'NONE', #9384, 1000.000000000000000 ) ;
#13774=CARTESIAN_POINT ( 'NONE',  ( 2.498001805406602216E-13, 3.000000000000002665, 6.000000000000158096 ) ) ;
#13776=DIRECTION ( 'NONE',  ( 1.000000000000000000, 1.771896121890576795E-14, 3.717264591378832268E-16 ) ) ;
#13781=ORIENTED_EDGE ( 'NONE', *, *, #8790, .F. ) ;
#13788=ORIENTED_EDGE ( 'NONE', *, *, #2235, .T. ) ;
#13793=CARTESIAN_POINT ( 'NONE',  ( 124.5000000000018332, -6.500000000000061284, -5.999999999999943157 ) ) ;
#13798=CARTESIAN_POINT ( 'NONE',  ( 66.26395429947838522, 0.000000000000000000, 6.500000000000144773 ) ) ;
#13810=EDGE_CURVE ( 'NONE', #13843, #11435, #17271, .T. ) ;
#13813=EDGE_LOOP ( 'NONE', ( #11954, #13588, #6902, #12474 ) ) ;
#13818=VECTOR ( 'NONE', #4933, 1000.000000000000000 ) ;
#13840=VECTOR ( 'NONE', #9294, 1000.000000000000000 ) ;
#13843=VERTEX_POINT ( 'NONE', #19818 ) ;
#13844=EDGE_CURVE ( 'NONE', #6978, #7176, #22176, .T. ) ;
#13845=ORIENTED_EDGE ( 'NONE', *, *, #16268, .T. ) ;
#13846=ADVANCED_FACE ( 'NONE', ( #16272 ), #14977, .T. ) ;
#13859=EDGE_CURVE ( 'NONE', #6130, #20921, #9690, .T. ) ;
#13893=DIRECTION ( 'NONE',  ( 3.032184104443272185E-30, 1.000000000000000000, -7.395570986447005381E-32 ) ) ;
#13896=ORIENTED_EDGE ( 'NONE', *, *, #17948, .T. ) ;
#13910=LINE ( 'NONE', #4961, #1889 ) ;
#13918=CYLINDRICAL_SURFACE ( 'NONE', #8194, 4.000000000000045297 ) ;
#13925=ORIENTED_EDGE ( 'NONE', *, *, #17478, .F. ) ;
#13931=ORIENTED_EDGE ( 'NONE', *, *, #14425, .T. ) ;
#13935=DIRECTION ( 'NONE',  ( -1.000000000000000000, 0.000000000000000000, -3.330669073875408978E-16 ) ) ;
#13937=AXIS2_PLACEMENT_3D ( 'NONE', #18211, #21848, #9610 ) ;
#13956=EDGE_CURVE ( 'NONE', #7176, #6978, #9419, .T. ) ;
#13968=ADVANCED_FACE ( 'NONE', ( #8279 ), #8655, .T. ) ;
#13969=VECTOR ( 'NONE', #7019, 1000.000000000000000 ) ;
#13970=AXIS2_PLACEMENT_3D ( 'NONE', #6651, #1138, #19230 ) ;
#13975=LINE ( 'NONE', #11628, #16442 ) ;
#13985=ORIENTED_EDGE ( 'NONE', *, *, #623, .F. ) ;
#13988=LINE ( 'NONE', #19634, #11400 ) ;
#13993=CARTESIAN_POINT ( 'NONE',  ( 87.68350880954425008, -11.67918431276149249, 6.500000000000179412 ) ) ;
#14005=DIRECTION ( 'NONE',  ( 1.000000000000000000, 2.699383410053119644E-30, 3.330669073875432643E-16 ) ) ;
#14020=DIRECTION ( 'NONE',  ( -4.003208021484906984E-16, 0.000000000000000000, 1.000000000000000000 ) ) ;
#14023=DIRECTION ( 'NONE',  ( -1.000000000000000000, -2.699383410053119644E-30, -3.330669073875432643E-16 ) ) ;
#14042=CARTESIAN_POINT ( 'NONE',  ( 108.2426266706970637, -13.52760560296359316, 5.999999999999984901 ) ) ;
#14044=AXIS2_PLACEMENT_3D ( 'NONE', #4663, #13725, #2895 ) ;
#14050=VERTEX_POINT ( 'NONE', #5090 ) ;
#14053=EDGE_CURVE ( 'NONE', #4929, #6497, #773, .T. ) ;
#14059=AXIS2_PLACEMENT_3D ( 'NONE', #18255, #14714, #15055 ) ;
#14062=CIRCLE ( 'NONE', #9918, 0.4999999999999984457 ) ;
#14067=PLANE ( 'NONE',  #22782 ) ;
#14075=DIRECTION ( 'NONE',  ( 1.000000000000000000, 0.000000000000000000, 4.336808689941968432E-16 ) ) ;
#14077=VERTEX_POINT ( 'NONE', #21094 ) ;
#14085=DIRECTION ( 'NONE',  ( -1.000000000000000000, 0.000000000000000000, -3.330669073875427220E-16 ) ) ;
#14093=CYLINDRICAL_SURFACE ( 'NONE', #299, 0.4999999999999987232 ) ;
#14103=ORIENTED_EDGE ( 'NONE', *, *, #15468, .T. ) ;
#14111=EDGE_CURVE ( 'NONE', #18843, #11516, #13910, .T. ) ;
#14119=LINE ( 'NONE', #15986, #15889 ) ;
#14135=ORIENTED_EDGE ( 'NONE', *, *, #18995, .F. ) ;
#14145=CARTESIAN_POINT ( 'NONE',  ( 119.5756419024615838, -6.500000000000005329, 6.000000000000158096 ) ) ;
#14146=DIRECTION ( 'NONE',  ( 1.850371707708574881E-14, 0.000000000000000000, 1.000000000000000000 ) ) ;
#14149=AXIS2_PLACEMENT_3D ( 'NONE', #6046, #13213, #13103 ) ;
#14160=ORIENTED_EDGE ( 'NONE', *, *, #16277, .T. ) ;
#14162=ORIENTED_EDGE ( 'NONE', *, *, #4491, .F. ) ;
#14176=FACE_BOUND ( 'NONE', #13733, .T. ) ;
#14181=DIRECTION ( 'NONE',  ( 0.000000000000000000, 0.000000000000000000, 1.000000000000000000 ) ) ;
#14191=EDGE_CURVE ( 'NONE', #3321, #13307, #19909, .T. ) ;
#14202=ORIENTED_EDGE ( 'NONE', *, *, #14851, .F. ) ;
#14206=DIRECTION ( 'NONE',  ( 0.000000000000000000, 0.000000000000000000, 1.000000000000000000 ) ) ;
#14219=LINE ( 'NONE', #14324, #8410 ) ;
#14223=EDGE_LOOP ( 'NONE', ( #13203, #4247, #21671, #1073 ) ) ;
#14232=DIRECTION ( 'NONE',  ( -4.003208021484906984E-16, 7.395570986447125806E-32, 1.000000000000000000 ) ) ;
#14275=CARTESIAN_POINT ( 'NONE',  ( 88.75737332930596324, -6.527605602963476805, 6.000000000000165201 ) ) ;
#14306=ORIENTED_EDGE ( 'NONE', *, *, #11403, .F. ) ;
#14314=DIRECTION ( 'NONE',  ( 3.032184104443272185E-30, 1.000000000000000000, -7.395570986447005381E-32 ) ) ;
#14324=CARTESIAN_POINT ( 'NONE',  ( 58.04599508018838350, 2.194061104857452982, 6.000000000000095923 ) ) ;
#14328=DIRECTION ( 'NONE',  ( 3.330669073875432643E-16, 4.437342591868153746E-31, -1.000000000000000000 ) ) ;
#14333=EDGE_LOOP ( 'NONE', ( #3115, #14600, #4462, #447 ) ) ;
#14344=CYLINDRICAL_SURFACE ( 'NONE', #16798, 7.000000000000075495 ) ;
#14358=VERTEX_POINT ( 'NONE', #4581 ) ;
#14379=CYLINDRICAL_SURFACE ( 'NONE', #4978, 0.4999999999999978351 ) ;
#14383=DIRECTION ( 'NONE',  ( 3.885780586188016830E-16, 4.437342591868156373E-31, -1.000000000000000000 ) ) ;
#14394=AXIS2_PLACEMENT_3D ( 'NONE', #21376, #17835, #18184 ) ;
#14395=VECTOR ( 'NONE', #6482, 1000.000000000000000 ) ;
#14414=CARTESIAN_POINT ( 'NONE',  ( 73.50000000000112266, -3.999999999999809042, 1.179611963664228824E-13 ) ) ;
#14422=ADVANCED_FACE ( 'NONE', ( #22127 ), #6018, .T. ) ;
#14425=EDGE_CURVE ( 'NONE', #4929, #17843, #15052, .T. ) ;
#14433=PLANE ( 'NONE',  #3176 ) ;
#14441=CARTESIAN_POINT ( 'NONE',  ( 6.500000000000005329, 1.665334536937734811E-13, 3.469446951953614189E-14 ) ) ;
#14445=CARTESIAN_POINT ( 'NONE',  ( 88.75737332930592061, -6.527605602963476805, -6.000000000000012434 ) ) ;
#14447=CARTESIAN_POINT ( 'NONE',  ( 86.02937988905580369, -9.453020409440155092, -6.499999999999943157 ) ) ;
#14449=CARTESIAN_POINT ( 'NONE',  ( 119.5756419024615411, -7.000000000000006217, 6.000000000000095923 ) ) ;
#14482=VECTOR ( 'NONE', #1529, 1000.000000000000000 ) ;
#14497=CARTESIAN_POINT ( 'NONE',  ( 113.0166151911345906, -11.64708151429785765, 6.000000000000067502 ) ) ;
#14502=CARTESIAN_POINT ( 'NONE',  ( 73.50000000000116529, -13.52760560296348302, -2.549999999999978062 ) ) ;
#14511=ORIENTED_EDGE ( 'NONE', *, *, #20482, .F. ) ;
#14523=ADVANCED_FACE ( 'NONE', ( #5179 ), #7072, .T. ) ;
#14525=CARTESIAN_POINT ( 'NONE',  ( 124.5000000000019185, -6.500000000000005329, 6.500000000000214051 ) ) ;
#14543=DIRECTION ( 'NONE',  ( 1.000000000000000000, 0.000000000000000000, 4.336808689941968432E-16 ) ) ;
#14548=ADVANCED_FACE ( 'NONE', ( #17521 ), #57, .T. ) ;
#14549=FACE_OUTER_BOUND ( 'NONE', #16228, .T. ) ;
#14553=CARTESIAN_POINT ( 'NONE',  ( 124.5000000000019469, -13.52760560296373171, 2.550000000000006040 ) ) ;
#14556=FACE_OUTER_BOUND ( 'NONE', #11061, .T. ) ;
#14571=DIRECTION ( 'NONE',  ( -1.000000000000000000, -5.598259082250514647E-17, -3.330669073875432643E-16 ) ) ;
#14573=EDGE_CURVE ( 'NONE', #5312, #16601, #7546, .T. ) ;
#14574=CIRCLE ( 'NONE', #1070, 0.5000000000000038858 ) ;
#14577=DIRECTION ( 'NONE',  ( 3.032184104443272185E-30, 1.000000000000000000, -7.395570986447005381E-32 ) ) ;
#14585=DIRECTION ( 'NONE',  ( 0.000000000000000000, 0.000000000000000000, 1.000000000000000000 ) ) ;
#14588=COLOUR_RGB ( '', 0.09019608, 0.27058824, 0.51372549) ;
#14600=ORIENTED_EDGE ( 'NONE', *, *, #8723, .F. ) ;
#14601=ORIENTED_EDGE ( 'NONE', *, *, #12844, .F. ) ;
#14606=DIRECTION ( 'NONE',  ( 3.885780586188016830E-16, 4.437342591868156373E-31, -1.000000000000000000 ) ) ;
#14620=ORIENTED_EDGE ( 'NONE', *, *, #14191, .T. ) ;
#14630=CARTESIAN_POINT ( 'NONE',  ( 124.5000000000017195, -4.500000000000003553, 6.500000000000123457 ) ) ;
#14632=EDGE_LOOP ( 'NONE', ( #6275, #13845, #22582, #23211 ) ) ;
#14633=DIRECTION ( 'NONE',  ( -3.330669073875432643E-16, -4.437342591868153746E-31, 1.000000000000000000 ) ) ;
#14668=CARTESIAN_POINT ( 'NONE',  ( 66.26395429947837101, -4.000000000000003553, 6.500000000000110134 ) ) ;
#14674=ORIENTED_EDGE ( 'NONE', *, *, #5530, .T. ) ;
#14685=DIRECTION ( 'NONE',  ( 3.032184104443272185E-30, 1.000000000000000000, -7.395570986447005381E-32 ) ) ;
#14686=EDGE_CURVE ( 'NONE', #9743, #700, #21840, .T. ) ;
#14691=VECTOR ( 'NONE', #13514, 1000.000000000000000 ) ;
#14702=AXIS2_PLACEMENT_3D ( 'NONE', #21868, #14023, #5088 ) ;
#14714=DIRECTION ( 'NONE',  ( 3.032184104443272185E-30, 1.000000000000000000, -7.395570986447005381E-32 ) ) ;
#14724=CIRCLE ( 'NONE', #2697, 4.000000000000045297 ) ;
#14728=ORIENTED_EDGE ( 'NONE', *, *, #15233, .T. ) ;
#14732=VERTEX_POINT ( 'NONE', #4446 ) ;
#14733=ORIENTED_EDGE ( 'NONE', *, *, #15426, .F. ) ;
#14739=DIRECTION ( 'NONE',  ( -0.6819983600625060260, -0.7313537016191635765, -6.106365041599011361E-16 ) ) ;
#14740=EDGE_LOOP ( 'NONE', ( #402, #18732, #11236, #9764 ) ) ;
#14745=DIRECTION ( 'NONE',  ( -0.7313537016191756779, 0.6819983600624930364, -4.478224685260177339E-16 ) ) ;
#14757=ORIENTED_EDGE ( 'NONE', *, *, #18050, .F. ) ;
#14766=CIRCLE ( 'NONE', #8390, 0.4999999999999990563 ) ;
#14769=EDGE_LOOP ( 'NONE', ( #4601, #14960, #6358, #2489 ) ) ;
#14773=DIRECTION ( 'NONE',  ( 3.885780586188016830E-16, 4.437342591868156373E-31, -1.000000000000000000 ) ) ;
#14775=EDGE_CURVE ( 'NONE', #11516, #13735, #2297, .T. ) ;
#14799=CARTESIAN_POINT ( 'NONE',  ( 57.15235153779114796, -1.074585193523325266, 6.000000000000185629 ) ) ;
#14800=ORIENTED_EDGE ( 'NONE', *, *, #9519, .T. ) ;
#14801=DIRECTION ( 'NONE',  ( -0.7313537016191745677, -0.6819983600624940356, -1.072890437865584285E-16 ) ) ;
#14803=CARTESIAN_POINT ( 'NONE',  ( 108.2426266706970637, -6.527605602963671316, -5.999999999999991118 ) ) ;
#14815=DIRECTION ( 'NONE',  ( 0.6819983600624998088, -0.7313537016191693496, 0.000000000000000000 ) ) ;
#14827=VERTEX_POINT ( 'NONE', #816 ) ;
#14838=ADVANCED_FACE ( 'NONE', ( #16783 ), #11275, .T. ) ;
#14840=LINE ( 'NONE', #21798, #13969 ) ;
#14851=EDGE_CURVE ( 'NONE', #12208, #4062, #22106, .T. ) ;
#14858=ORIENTED_EDGE ( 'NONE', *, *, #2062, .T. ) ;
#14861=ORIENTED_EDGE ( 'NONE', *, *, #6967, .F. ) ;
#14866=CARTESIAN_POINT ( 'NONE',  ( 124.5000000000019469, -7.000000000000062172, 2.081668171172168513E-14 ) ) ;
#14871=DIRECTION ( 'NONE',  ( -0.7313537016191767881, -0.6819983600624918152, -4.403559511741033569E-16 ) ) ;
#14883=ORIENTED_EDGE ( 'NONE', *, *, #44, .F. ) ;
#14884=EDGE_LOOP ( 'NONE', ( #11460, #2821, #6871, #18074 ) ) ;
#14901=LINE ( 'NONE', #14553, #13756 ) ;
#14934=VECTOR ( 'NONE', #18109, 1000.000000000000000 ) ;
#14949=DIRECTION ( 'NONE',  ( -3.885780586188016830E-16, -4.437342591868156373E-31, 1.000000000000000000 ) ) ;
#14960=ORIENTED_EDGE ( 'NONE', *, *, #10946, .F. ) ;
#14969=DIRECTION ( 'NONE',  ( -0.7313537016191755669, 0.6819983600624931475, -2.390712761620034777E-15 ) ) ;
#14973=CYLINDRICAL_SURFACE ( 'NONE', #15569, 0.5000000000000038858 ) ;
#14977=CYLINDRICAL_SURFACE ( 'NONE', #22924, 0.5000000000000038858 ) ;
#14982=ADVANCED_FACE ( 'NONE', ( #7274 ), #16926, .T. ) ;
#14990=AXIS2_PLACEMENT_3D ( 'NONE', #10768, #1829, #9013 ) ;
#14994=EDGE_LOOP ( 'NONE', ( #2787, #15304, #5919, #1156 ) ) ;
#15012=PLANE ( 'NONE',  #2381 ) ;
#15016=ORIENTED_EDGE ( 'NONE', *, *, #2183, .T. ) ;
#15037=DIRECTION ( 'NONE',  ( -1.000000000000000000, 0.000000000000000000, -4.336808689941968432E-16 ) ) ;
#15042=EDGE_LOOP ( 'NONE', ( #14601, #15824, #3948, #18943 ) ) ;
#15052=LINE ( 'NONE', #22244, #4897 ) ;
#15055=DIRECTION ( 'NONE',  ( 0.000000000000000000, 0.000000000000000000, 1.000000000000000000 ) ) ;
#15068=ORIENTED_EDGE ( 'NONE', *, *, #3043, .T. ) ;
#15075=ORIENTED_EDGE ( 'NONE', *, *, #10734, .T. ) ;
#15077=DIRECTION ( 'NONE',  ( 1.000000000000000000, 2.699383410053119644E-30, 3.330669073875432643E-16 ) ) ;
#15082=CARTESIAN_POINT ( 'NONE',  ( 108.2426266706970353, -13.52760560296359316, -6.000000000000019540 ) ) ;
#15090=DIRECTION ( 'NONE',  ( -1.000000000000000000, -2.699383410053121045E-30, -3.717264591378832268E-16 ) ) ;
#15113=AXIS2_PLACEMENT_3D ( 'NONE', #23226, #7113, #1795 ) ;
#15115=CYLINDRICAL_SURFACE ( 'NONE', #9344, 7.000000000000075495 ) ;
#15121=ADVANCED_FACE ( 'NONE', ( #16989 ), #18427, .T. ) ;
#15160=CARTESIAN_POINT ( 'NONE',  ( 124.5000000000019469, -13.52760560296373171, -6.938893903907228378E-15 ) ) ;
#15161=AXIS2_PLACEMENT_3D ( 'NONE', #21606, #18070, #9237 ) ;
#15180=CARTESIAN_POINT ( 'NONE',  ( 113.0166151911346475, -11.64708151429785765, -6.000000000000012434 ) ) ;
#15181=DIRECTION ( 'NONE',  ( 0.000000000000000000, 0.000000000000000000, 1.000000000000000000 ) ) ;
#15201=DIRECTION ( 'NONE',  ( 3.330669073875432643E-16, 4.437342591868153746E-31, -1.000000000000000000 ) ) ;
#15210=DIRECTION ( 'NONE',  ( 1.000000000000000000, -1.847414967615758933E-47, 3.885780586188017323E-16 ) ) ;
#15216=ORIENTED_EDGE ( 'NONE', *, *, #19333, .T. ) ;
#15233=EDGE_CURVE ( 'NONE', #21954, #20178, #16940, .T. ) ;
#15235=CARTESIAN_POINT ( 'NONE',  ( 124.5000000000017764, -4.500000000000003553, 6.000000000000116351 ) ) ;
#15254=CARTESIAN_POINT ( 'NONE',  ( 54.42435809754106657, -4.000000000000003553, 6.000000000000136779 ) ) ;
#15263=ADVANCED_FACE ( 'NONE', ( #8192 ), #4878, .T. ) ;
#15271=AXIS2_PLACEMENT_3D ( 'NONE', #9861, #935, #8093 ) ;
#15294=ADVANCED_FACE ( 'NONE', ( #23009 ), #18840, .T. ) ;
#15297=CARTESIAN_POINT ( 'NONE',  ( 77.42435809754130105, -10.99999999999981526, 6.000000000000123457 ) ) ;
#15303=LINE ( 'NONE', #4243, #1769 ) ;
#15304=ORIENTED_EDGE ( 'NONE', *, *, #7206, .F. ) ;
#15316=VECTOR ( 'NONE', #1000, 1000.000000000000000 ) ;
#15321=EDGE_CURVE ( 'NONE', #14050, #15515, #20355, .T. ) ;
#15348=DIRECTION ( 'NONE',  ( -0.6819983600624981435, -0.7313537016191709039, 0.000000000000000000 ) ) ;
#15357=CARTESIAN_POINT ( 'NONE',  ( 124.5000000000019469, -6.500000000000061284, 4.857225732735059864E-14 ) ) ;
#15360=DIRECTION ( 'NONE',  ( 0.000000000000000000, 0.000000000000000000, 1.000000000000000000 ) ) ;
#15372=CIRCLE ( 'NONE', #11246, 4.500000000000045297 ) ;
#15378=CARTESIAN_POINT ( 'NONE',  ( 6.500000000000227374, 1.665334536937734811E-13, 6.000000000000213163 ) ) ;
#15379=DIRECTION ( 'NONE',  ( -3.885780586188016830E-16, -4.437342591868156373E-31, 1.000000000000000000 ) ) ;
#15380=CIRCLE ( 'NONE', #9001, 0.5000000000000038858 ) ;
#15387=DIRECTION ( 'NONE',  ( 3.032184104443272185E-30, 1.000000000000000000, -7.395570986447005381E-32 ) ) ;
#15396=ORIENTED_EDGE ( 'NONE', *, *, #16415, .F. ) ;
#15406=CARTESIAN_POINT ( 'NONE',  ( 6.500000000000227374, 0.5000000000001669775, 6.000000000000213163 ) ) ;
#15426=EDGE_CURVE ( 'NONE', #5256, #13332, #18859, .T. ) ;
#15428=AXIS2_PLACEMENT_3D ( 'NONE', #15522, #22718, #6598 ) ;
#15437=CARTESIAN_POINT ( 'NONE',  ( 88.75737332930594903, -13.52760560296348302, 6.000000000000130562 ) ) ;
#15445=AXIS2_PLACEMENT_3D ( 'NONE', #15357, #18780, #8073 ) ;
#15451=EDGE_CURVE ( 'NONE', #12056, #11543, #14840, .T. ) ;
#15461=EDGE_LOOP ( 'NONE', ( #15075, #15677, #20734, #20159 ) ) ;
#15468=EDGE_CURVE ( 'NONE', #273, #14077, #262, .T. ) ;
#15470=DIRECTION ( 'NONE',  ( 0.000000000000000000, 0.000000000000000000, 1.000000000000000000 ) ) ;
#15492=DIRECTION ( 'NONE',  ( -3.885780586188016830E-16, -4.437342591868156373E-31, 1.000000000000000000 ) ) ;
#15493=DIRECTION ( 'NONE',  ( 3.885780586188016830E-16, 4.437342591868156373E-31, -1.000000000000000000 ) ) ;
#15510=EDGE_LOOP ( 'NONE', ( #9455, #9832, #6210, #19078 ) ) ;
#15513=AXIS2_PLACEMENT_3D ( 'NONE', #8727, #10939, #14020 ) ;
#15515=VERTEX_POINT ( 'NONE', #15180 ) ;
#15518=DIRECTION ( 'NONE',  ( -0.6819983600625055820, -0.7313537016191637985, -4.996142016973858765E-16 ) ) ;
#15522=CARTESIAN_POINT ( 'NONE',  ( 57.70499590015723612, 1.828384254047854540, 6.000000000000136779 ) ) ;
#15524=ADVANCED_FACE ( 'NONE', ( #16813 ), #13314, .T. ) ;
#15531=CIRCLE ( 'NONE', #6531, 7.000000000000075495 ) ;
#15534=VECTOR ( 'NONE', #17661, 1000.000000000000000 ) ;
#15546=CIRCLE ( 'NONE', #6917, 0.4999999999999993894 ) ;
#15547=EDGE_LOOP ( 'NONE', ( #2462, #12886, #3549, #23186 ) ) ;
#15551=EDGE_CURVE ( 'NONE', #4929, #4634, #20757, .T. ) ;
#15569=AXIS2_PLACEMENT_3D ( 'NONE', #20284, #20392, #6276 ) ;
#15572=ORIENTED_EDGE ( 'NONE', *, *, #9406, .T. ) ;
#15574=SHAPE_REPRESENTATION ( 'Half Handle', ( #22115 ), #712 ) ;
#15577=ADVANCED_FACE ( 'NONE', ( #4587 ), #11767, .T. ) ;
#15578=VERTEX_POINT ( 'NONE', #5752 ) ;
#15582=ORIENTED_EDGE ( 'NONE', *, *, #5054, .F. ) ;
#15592=EDGE_CURVE ( 'NONE', #18277, #14827, #694, .T. ) ;
#15595=ORIENTED_EDGE ( 'NONE', *, *, #8990, .F. ) ;
#15604=ORIENTED_EDGE ( 'NONE', *, *, #5341, .F. ) ;
#15607=ORIENTED_EDGE ( 'NONE', *, *, #4874, .F. ) ;
#15613=DIRECTION ( 'NONE',  ( -1.000000000000000000, -2.699383410053119644E-30, -3.330669073875432643E-16 ) ) ;
#15627=TOROIDAL_SURFACE ( 'NONE', #4734, 4.500000000000000888, 0.5000000000000000000 ) ;
#15636=VERTEX_POINT ( 'NONE', #18563 ) ;
#15639=DIRECTION ( 'NONE',  ( 3.032184104443272185E-30, 1.000000000000000000, -7.395570986447005381E-32 ) ) ;
#15643=DIRECTION ( 'NONE',  ( -3.885780586188016830E-16, -4.437342591868156373E-31, 1.000000000000000000 ) ) ;
#15653=VERTEX_POINT ( 'NONE', #14799 ) ;
#15663=DIRECTION ( 'NONE',  ( 3.885780586188016830E-16, 4.437342591868156373E-31, -1.000000000000000000 ) ) ;
#15674=AXIS2_PLACEMENT_3D ( 'NONE', #3814, #10987, #18185 ) ;
#15676=ADVANCED_FACE ( 'NONE', ( #20220 ), #7513, .T. ) ;
#15677=ORIENTED_EDGE ( 'NONE', *, *, #7242, .T. ) ;
#15679=VECTOR ( 'NONE', #21690, 1000.000000000000000 ) ;
#15700=FACE_OUTER_BOUND ( 'NONE', #19724, .T. ) ;
#15710=DIRECTION ( 'NONE',  ( -1.000000000000000000, -2.699383410053119644E-30, -3.330669073875432643E-16 ) ) ;
#15712=DIRECTION ( 'NONE',  ( -0.7313537016191730133, 0.6819983600624958120, -5.924440990721418971E-17 ) ) ;
#15717=ORIENTED_EDGE ( 'NONE', *, *, #11582, .F. ) ;
#15727=CARTESIAN_POINT ( 'NONE',  ( 119.5756419024615553, -11.00000000000006573, 6.500000000000012434 ) ) ;
#15729=VECTOR ( 'NONE', #8196, 1000.000000000000000 ) ;
#15731=DIRECTION ( 'NONE',  ( 1.000000000000000000, 2.699383410053118943E-30, 2.668805347656595124E-16 ) ) ;
#15736=DIRECTION ( 'NONE',  ( 3.885780586188016830E-16, 4.437342591868156373E-31, -1.000000000000000000 ) ) ;
#15739=VERTEX_POINT ( 'NONE', #16548 ) ;
#15740=AXIS2_PLACEMENT_3D ( 'NONE', #18296, #21833, #11110 ) ;
#15774=CARTESIAN_POINT ( 'NONE',  ( 108.2426266706971205, -10.52760560296367487, -6.500000000000075495 ) ) ;
#15777=AXIS2_PLACEMENT_3D ( 'NONE', #6048, #1111, #11443 ) ;
#15778=DIRECTION ( 'NONE',  ( -3.241725282392603095E-30, -1.000000000000000000, 2.218671295934100958E-31 ) ) ;
#15794=ORIENTED_EDGE ( 'NONE', *, *, #4802, .T. ) ;
#15797=ORIENTED_EDGE ( 'NONE', *, *, #2157, .T. ) ;
#15798=EDGE_LOOP ( 'NONE', ( #18270, #3241, #12258, #3460 ) ) ;
#15804=DIRECTION ( 'NONE',  ( -1.000000000000000000, -2.699383410053119644E-30, -3.330669073875432643E-16 ) ) ;
#15810=DIRECTION ( 'NONE',  ( -0.6819983600625081355, -0.7313537016191615781, 0.000000000000000000 ) ) ;
#15815=CARTESIAN_POINT ( 'NONE',  ( 77.42435809754130105, -10.99999999999981526, 6.000000000000123457 ) ) ;
#15817=EDGE_CURVE ( 'NONE', #22680, #19728, #3977, .T. ) ;
#15819=CARTESIAN_POINT ( 'NONE',  ( 114.8016533820240568, -5.880524088665878502, -6.499999999999970690 ) ) ;
#15824=ORIENTED_EDGE ( 'NONE', *, *, #12556, .T. ) ;
#15827=CARTESIAN_POINT ( 'NONE',  ( 65.19008977971681418, -5.151578709798015687, 6.500000000000179412 ) ) ;
#15845=ADVANCED_FACE ( 'NONE', ( #350 ), #19428, .T. ) ;
#15862=DIRECTION ( 'NONE',  ( 1.000000000000000000, 0.000000000000000000, 4.336808689941968432E-16 ) ) ;
#15886=DIRECTION ( 'NONE',  ( 3.885780586188016830E-16, 4.437342591868156373E-31, -1.000000000000000000 ) ) ;
#15887=AXIS2_PLACEMENT_3D ( 'NONE', #9759, #17264, #1170 ) ;
#15889=VECTOR ( 'NONE', #19292, 1000.000000000000114 ) ;
#15895=AXIS2_PLACEMENT_3D ( 'NONE', #13793, #16008, #19087 ) ;
#15898=DIRECTION ( 'NONE',  ( -1.000000000000000000, 1.865174681370276872E-14, -3.854941057726193231E-16 ) ) ;
#15916=VERTEX_POINT ( 'NONE', #13164 ) ;
#15918=DIRECTION ( 'NONE',  ( 0.000000000000000000, 1.000000000000000000, 0.000000000000000000 ) ) ;
#15919=FACE_OUTER_BOUND ( 'NONE', #22063, .T. ) ;
#15925=CARTESIAN_POINT ( 'NONE',  ( 54.42435809754118736, 2.999999999999947153, -6.499999999999922728 ) ) ;
#15930=CARTESIAN_POINT ( 'NONE',  ( 54.42435809754113052, -4.000000000000003553, -6.000000000000012434 ) ) ;
#15936=CARTESIAN_POINT ( 'NONE',  ( 66.26395429947839943, -7.000000000000006217, -6.000000000000060396 ) ) ;
#15938=CARTESIAN_POINT ( 'NONE',  ( 108.2426266706970353, -13.02760560296359316, -6.000000000000019540 ) ) ;
#15944=EDGE_LOOP ( 'NONE', ( #14674, #16174, #4406, #15396 ) ) ;
#15967=ADVANCED_FACE ( 'NONE', ( #16779 ), #12075, .T. ) ;
#15983=EDGE_CURVE ( 'NONE', #10216, #522, #831, .T. ) ;
#15986=CARTESIAN_POINT ( 'NONE',  ( 78.36587326203826365, -2.990348597579628454, -6.499999999999984901 ) ) ;
#16008=DIRECTION ( 'NONE',  ( -1.000000000000000000, -2.699383410053119644E-30, -3.330669073875432643E-16 ) ) ;
#16024=DIRECTION ( 'NONE',  ( 1.000000000000000000, 2.699383410053119644E-30, 3.330669073875432643E-16 ) ) ;
#16052=DIRECTION ( 'NONE',  ( 0.000000000000000000, 0.000000000000000000, 1.000000000000000000 ) ) ;
#16056=VECTOR ( 'NONE', #14685, 1000.000000000000000 ) ;
#16059=VERTEX_POINT ( 'NONE', #13626 ) ;
#16070=AXIS2_PLACEMENT_3D ( 'NONE', #17256, #17024, #10323 ) ;
#16080=EDGE_CURVE ( 'NONE', #15636, #19862, #11340, .T. ) ;
#16096=DIRECTION ( 'NONE',  ( -0.7313537016191746787, 0.6819983600624941467, 5.177789255530095281E-17 ) ) ;
#16104=AXIS2_PLACEMENT_3D ( 'NONE', #21721, #5720, #13123 ) ;
#16107=( NAMED_UNIT ( * ) PLANE_ANGLE_UNIT ( ) SI_UNIT ( $, .RADIAN. ) );
#16118=VERTEX_POINT ( 'NONE', #10441 ) ;
#16127=EDGE_CURVE ( 'NONE', #5606, #2826, #1955, .T. ) ;
#16151=VERTEX_POINT ( 'NONE', #3721 ) ;
#16152=ORIENTED_EDGE ( 'NONE', *, *, #2937, .T. ) ;
#16162=AXIS2_PLACEMENT_3D ( 'NONE', #11902, #19089, #17310 ) ;
#16164=ADVANCED_FACE ( 'NONE', ( #317 ), #1839, .F. ) ;
#16174=ORIENTED_EDGE ( 'NONE', *, *, #16127, .F. ) ;
#16183=DIRECTION ( 'NONE',  ( -3.032184104443272185E-30, -1.000000000000000000, 7.395570986447005381E-32 ) ) ;
#16186=DIRECTION ( 'NONE',  ( -1.000000000000000000, -2.699383410053119644E-30, -3.330669073875432643E-16 ) ) ;
#16196=ORIENTED_EDGE ( 'NONE', *, *, #626, .T. ) ;
#16202=DIRECTION ( 'NONE',  ( 0.6819983600625060260, 0.7313537016191635765, 6.106365041599011361E-16 ) ) ;
#16205=CARTESIAN_POINT ( 'NONE',  ( 124.5000000000019469, -4.000000000000058620, -2.549999999999978506 ) ) ;
#16225=AXIS2_PLACEMENT_3D ( 'NONE', #5968, #16410, #7380 ) ;
#16228=EDGE_LOOP ( 'NONE', ( #12205, #22528, #21084, #8495 ) ) ;
#16233=CIRCLE ( 'NONE', #12878, 6.500000000000075495 ) ;
#16236=DIRECTION ( 'NONE',  ( 3.032184104443271834E-30, 1.000000000000000000, 4.437342591868167759E-31 ) ) ;
#16259=ORIENTED_EDGE ( 'NONE', *, *, #22021, .F. ) ;
#16268=EDGE_CURVE ( 'NONE', #22610, #18277, #12850, .T. ) ;
#16272=FACE_OUTER_BOUND ( 'NONE', #5265, .T. ) ;
#16275=DIRECTION ( 'NONE',  ( 0.6819983600625060260, 0.7313537016191635765, 6.106365041599011361E-16 ) ) ;
#16277=EDGE_CURVE ( 'NONE', #2970, #10913, #14724, .T. ) ;
#16291=ORIENTED_EDGE ( 'NONE', *, *, #3338, .F. ) ;
#16295=ADVANCED_FACE ( 'NONE', ( #13243 ), #2653, .T. ) ;
#16297=ADVANCED_FACE ( 'NONE', ( #13366 ), #5352, .T. ) ;
#16302=CIRCLE ( 'NONE', #1294, 0.5000000000000038858 ) ;
#16305=TOROIDAL_SURFACE ( 'NONE', #6182, 6.500000000000000888, 0.5000000000000000000 ) ;
#16314=DIRECTION ( 'NONE',  ( -1.000000000000000000, -2.699383410053119644E-30, -3.330669073875432643E-16 ) ) ;
#16315=DIRECTION ( 'NONE',  ( -3.885780586188016830E-16, -4.437342591868156373E-31, 1.000000000000000000 ) ) ;
#16319=AXIS2_PLACEMENT_3D ( 'NONE', #22392, #22617, #17194 ) ;
#16325=ORIENTED_EDGE ( 'NONE', *, *, #2829, .F. ) ;
#16332=AXIS2_PLACEMENT_3D ( 'NONE', #1106, #2855, #6396 ) ;
#16362=DIRECTION ( 'NONE',  ( -0.7313537016191742346, 0.6819983600624944797, 1.072890437865585765E-16 ) ) ;
#16389=CARTESIAN_POINT ( 'NONE',  ( 54.42435809754106657, -4.000000000000003553, 6.000000000000136779 ) ) ;
#16399=ORIENTED_EDGE ( 'NONE', *, *, #1522, .F. ) ;
#16400=( GEOMETRIC_REPRESENTATION_CONTEXT ( 3 ) GLOBAL_UNCERTAINTY_ASSIGNED_CONTEXT ( ( #2493 ) ) GLOBAL_UNIT_ASSIGNED_CONTEXT ( ( #11423, #18608, #18716 ) ) REPRESENTATION_CONTEXT ( 'NONE', 'WORKASPACE' ) );
#16410=DIRECTION ( 'NONE',  ( -0.7313537016191772322, -0.6819983600624914821, -3.241477906037841845E-14 ) ) ;
#16415=EDGE_CURVE ( 'NONE', #4164, #11689, #3100, .T. ) ;
#16428=VECTOR ( 'NONE', #20529, 1000.000000000000000 ) ;
#16433=AXIS2_PLACEMENT_3D ( 'NONE', #11807, #20765, #8406 ) ;
#16435=DIRECTION ( 'NONE',  ( 0.6819983600624998088, -0.7313537016191693496, 0.000000000000000000 ) ) ;
#16436=ORIENTED_EDGE ( 'NONE', *, *, #10707, .T. ) ;
#16442=VECTOR ( 'NONE', #2934, 1000.000000000000000 ) ;
#16452=CARTESIAN_POINT ( 'NONE',  ( 54.42435809754109499, 0.4999999999999449329, 6.500000000000144773 ) ) ;
#16465=ORIENTED_EDGE ( 'NONE', *, *, #9406, .F. ) ;
#16499=DIRECTION ( 'NONE',  ( 3.885780586188016830E-16, 4.437342591868156373E-31, -1.000000000000000000 ) ) ;
#16512=AXIS2_PLACEMENT_3D ( 'NONE', #21370, #19351, #71 ) ;
#16524=CARTESIAN_POINT ( 'NONE',  ( 116.8476484622115805, -8.074585193523331483, -5.999999999999956479 ) ) ;
#16538=AXIS2_PLACEMENT_3D ( 'NONE', #7891, #13422, #20603 ) ;
#16542=EDGE_CURVE ( 'NONE', #8580, #4606, #17694, .T. ) ;
#16546=CARTESIAN_POINT ( 'NONE',  ( 88.75737332930596324, -6.527605602963476805, 6.000000000000165201 ) ) ;
#16548=CARTESIAN_POINT ( 'NONE',  ( 83.98338480886826574, -11.64708151429766403, -6.000000000000019540 ) ) ;
#16553=CARTESIAN_POINT ( 'NONE',  ( 80.49335071782269324, -7.708908342713566064, -5.999999999999998224 ) ) ;
#16561=DIRECTION ( 'NONE',  ( 3.032184104443272185E-30, 1.000000000000000000, -7.395570986447005381E-32 ) ) ;
#16573=ORIENTED_EDGE ( 'NONE', *, *, #12263, .T. ) ;
#16580=DIRECTION ( 'NONE',  ( -1.000000000000000000, 4.795271322878693306E-14, -3.717264591378832268E-16 ) ) ;
#16581=DIRECTION ( 'NONE',  ( -1.000000000000000000, -2.699383410053119644E-30, -3.330669073875432643E-16 ) ) ;
#16587=AXIS2_PLACEMENT_3D ( 'NONE', #7743, #7979, #11615 ) ;
#16591=VERTEX_POINT ( 'NONE', #5116 ) ;
#16601=VERTEX_POINT ( 'NONE', #8883 ) ;
#16602=CARTESIAN_POINT ( 'NONE',  ( 86.02937988905583211, -9.453020409440155092, 6.000000000000165201 ) ) ;
#16608=DIRECTION ( 'NONE',  ( 3.885780586188016830E-16, 4.437342591868156373E-31, -1.000000000000000000 ) ) ;
#16614=AXIS2_PLACEMENT_3D ( 'NONE', #573, #2213, #9167 ) ;
#16624=CIRCLE ( 'NONE', #14394, 0.5000000000000033307 ) ;
#16633=AXIS2_PLACEMENT_3D ( 'NONE', #9796, #14969, #18393 ) ;
#16646=AXIS2_PLACEMENT_3D ( 'NONE', #18342, #14577, #21764 ) ;
#16649=CIRCLE ( 'NONE', #21936, 7.000000000000075495 ) ;
#16650=CIRCLE ( 'NONE', #17801, 0.5000000000000038858 ) ;
#16663=AXIS2_PLACEMENT_3D ( 'NONE', #10635, #3363, #15918 ) ;
#16670=FACE_OUTER_BOUND ( 'NONE', #9335, .T. ) ;
#16675=FACE_OUTER_BOUND ( 'NONE', #22263, .T. ) ;
#16680=CARTESIAN_POINT ( 'NONE',  ( 83.98338480886830837, -11.64708151429766403, 6.000000000000136779 ) ) ;
#16681=LINE ( 'NONE', #590, #13840 ) ;
#16683=FACE_OUTER_BOUND ( 'NONE', #10934, .T. ) ;
#16691=ORIENTED_EDGE ( 'NONE', *, *, #6611, .F. ) ;
#16693=CARTESIAN_POINT ( 'NONE',  ( 88.75737332930596324, -13.02760560296348302, -6.499999999999964473 ) ) ;
#16704=CARTESIAN_POINT ( 'NONE',  ( 115.1426525620552468, -6.246200939475476943, -6.499999999999950262 ) ) ;
#16717=EDGE_LOOP ( 'NONE', ( #20390, #15604, #21556, #14733 ) ) ;
#16749=ORIENTED_EDGE ( 'NONE', *, *, #11324, .T. ) ;
#16756=DIRECTION ( 'NONE',  ( 3.032184104443272185E-30, 1.000000000000000000, -7.395570986447005381E-32 ) ) ;
#16768=CIRCLE ( 'NONE', #5137, 0.4999999999999990563 ) ;
#16770=EDGE_LOOP ( 'NONE', ( #1409, #4028, #2724, #11599 ) ) ;
#16775=VERTEX_POINT ( 'NONE', #17311 ) ;
#16779=FACE_OUTER_BOUND ( 'NONE', #1269, .T. ) ;
#16783=FACE_OUTER_BOUND ( 'NONE', #15461, .T. ) ;
#16789=CYLINDRICAL_SURFACE ( 'NONE', #4443, 4.000000000000045297 ) ;
#16798=AXIS2_PLACEMENT_3D ( 'NONE', #8828, #17640, #3749 ) ;
#16799=AXIS2_PLACEMENT_3D ( 'NONE', #3682, #9326, #1798 ) ;
#16809=CIRCLE ( 'NONE', #3672, 6.500000000000075495 ) ;
#16813=FACE_OUTER_BOUND ( 'NONE', #17506, .T. ) ;
#16830=UNCERTAINTY_MEASURE_WITH_UNIT (LENGTH_MEASURE( 1.000000000000000082E-05 ), #5192, 'distance_accuracy_value', 'NONE');
#16837=DIRECTION ( 'NONE',  ( -3.241725282392603095E-30, -1.000000000000000000, 2.218671295934100958E-31 ) ) ;
#16859=PLANE ( 'NONE',  #12331 ) ;
#16866=ORIENTED_EDGE ( 'NONE', *, *, #2786, .T. ) ;
#16867=VERTEX_POINT ( 'NONE', #18031 ) ;
#16889=DIRECTION ( 'NONE',  ( -1.000000000000000000, -2.699383410053119644E-30, -3.330669073875432643E-16 ) ) ;
#16898=VERTEX_POINT ( 'NONE', #23219 ) ;
#16905=FACE_OUTER_BOUND ( 'NONE', #14223, .T. ) ;
#16912=LINE ( 'NONE', #12816, #9325 ) ;
#16919=ADVANCED_FACE ( 'NONE', ( #3671, #1894 ), #5212, .T. ) ;
#16926=TOROIDAL_SURFACE ( 'NONE', #19212, 4.500000000000000888, 0.5000000000000000000 ) ;
#16930=CARTESIAN_POINT ( 'NONE',  ( 119.5756419024615838, -11.00000000000006573, -6.000000000000116351 ) ) ;
#16932=CARTESIAN_POINT ( 'NONE',  ( 119.5756419024615269, -11.00000000000006573, 6.000000000000081712 ) ) ;
#16933=CARTESIAN_POINT ( 'NONE',  ( 6.500000000000283329, 2.500000000000168754, -5.999999999999943157 ) ) ;
#16940=CIRCLE ( 'NONE', #18470, 0.5000000000000038858 ) ;
#16943=ORIENTED_EDGE ( 'NONE', *, *, #9860, .F. ) ;
#16951=EDGE_LOOP ( 'NONE', ( #17216, #982 ) ) ;
#16957=CARTESIAN_POINT ( 'NONE',  ( 86.00000000000117950, -11.02760560296348125, 6.000000000000054179 ) ) ;
#16958=EDGE_CURVE ( 'NONE', #3270, #16867, #18145, .T. ) ;
#16964=DIRECTION ( 'NONE',  ( 3.885780586188016830E-16, 4.437342591868156373E-31, -1.000000000000000000 ) ) ;
#16978=AXIS2_PLACEMENT_3D ( 'NONE', #10442, #3616, #6924 ) ;
#16985=DIRECTION ( 'NONE',  ( 1.000000000000000000, -1.847414967615758933E-47, 3.885780586188017323E-16 ) ) ;
#16989=FACE_OUTER_BOUND ( 'NONE', #9850, .T. ) ;
#17000=AXIS2_PLACEMENT_3D ( 'NONE', #148, #17789, #10490 ) ;
#17024=DIRECTION ( 'NONE',  ( -0.6819983600624940356, 0.7313537016191746787, 1.110361430785838977E-16 ) ) ;
#17028=CARTESIAN_POINT ( 'NONE',  ( 83.98338480886823731, -11.64708151429766403, 6.500000000000117240 ) ) ;
#17040=ORIENTED_EDGE ( 'NONE', *, *, #5182, .F. ) ;
#17061=LINE ( 'NONE', #10022, #22808 ) ;
#17068=ORIENTED_EDGE ( 'NONE', *, *, #6203, .T. ) ;
#17104=CARTESIAN_POINT ( 'NONE',  ( 119.5756419024615838, -11.00000000000006573, -6.000000000000116351 ) ) ;
#17118=ADVANCED_FACE ( 'NONE', ( #22128 ), #6019, .F. ) ;
#17125=ORIENTED_EDGE ( 'NONE', *, *, #4491, .T. ) ;
#17128=ORIENTED_EDGE ( 'NONE', *, *, #12716, .F. ) ;
#17131=ORIENTED_EDGE ( 'NONE', *, *, #1210, .T. ) ;
#17138=DIRECTION ( 'NONE',  ( 0.000000000000000000, 0.000000000000000000, 1.000000000000000000 ) ) ;
#17141=CARTESIAN_POINT ( 'NONE',  ( 59.19834661797866460, 2.499999999999946709, 6.500000000000130562 ) ) ;
#17169=CARTESIAN_POINT ( 'NONE',  ( 115.1426525620553036, -6.246200939475421876, 6.500000000000137668 ) ) ;
#17178=LINE ( 'NONE', #22138, #20242 ) ;
#17182=ORIENTED_EDGE ( 'NONE', *, *, #8529, .F. ) ;
#17194=DIRECTION ( 'NONE',  ( 1.000000000000000000, 0.000000000000000000, 2.668805347656595124E-16 ) ) ;
#17216=ORIENTED_EDGE ( 'NONE', *, *, #1173, .T. ) ;
#17218=TOROIDAL_SURFACE ( 'NONE', #3710, 6.500000000000000888, 0.5000000000000000000 ) ;
#17220=VECTOR ( 'NONE', #7472, 1000.000000000000000 ) ;
#17222=EDGE_CURVE ( 'NONE', #22610, #13451, #3853, .T. ) ;
#17234=DIRECTION ( 'NONE',  ( -1.000000000000000000, -2.699383410053119644E-30, -3.330669073875432643E-16 ) ) ;
#17247=EDGE_CURVE ( 'NONE', #9421, #18277, #19656, .T. ) ;
#17256=CARTESIAN_POINT ( 'NONE',  ( 108.9540049198142100, -11.33354449810597409, 6.500000000000040856 ) ) ;
#17264=DIRECTION ( 'NONE',  ( -3.330669073875432643E-16, -4.437342591868153746E-31, 1.000000000000000000 ) ) ;
#17270=EDGE_CURVE ( 'NONE', #18651, #13735, #6599, .T. ) ;
#17271=CIRCLE ( 'NONE', #386, 0.5000000000000034417 ) ;
#17300=ORIENTED_EDGE ( 'NONE', *, *, #9307, .F. ) ;
#17310=DIRECTION ( 'NONE',  ( 1.000000000000000000, 2.699383410053120695E-30, 3.885780586188017323E-16 ) ) ;
#17311=CARTESIAN_POINT ( 'NONE',  ( 111.3116192909783138, -9.818697260249948044, -6.500000000000047073 ) ) ;
#17314=EDGE_CURVE ( 'NONE', #20860, #3634, #14119, .T. ) ;
#17326=EDGE_LOOP ( 'NONE', ( #12895, #18592, #1469, #17682 ) ) ;
#17345=CARTESIAN_POINT ( 'NONE',  ( 112.6756160111033722, -11.28140466348826010, -6.000000000000047073 ) ) ;
#17346=DIRECTION ( 'NONE',  ( -0.7313537016191715701, 0.6819983600624975884, 1.072890437865588353E-16 ) ) ;
#17347=CARTESIAN_POINT ( 'NONE',  ( 57.15235153779114796, -1.074585193523325266, 6.000000000000185629 ) ) ;
#17355=CARTESIAN_POINT ( 'NONE',  ( 6.500000000000339284, 0.5000000000001392220, -6.499999999999957367 ) ) ;
#17364=ORIENTED_EDGE ( 'NONE', *, *, #22216, .F. ) ;
#17377=CYLINDRICAL_SURFACE ( 'NONE', #17564, 0.5000000000000038858 ) ;
#17384=CIRCLE ( 'NONE', #12937, 0.4999999999999990563 ) ;
#17385=VECTOR ( 'NONE', #20955, 1000.000000000000000 ) ;
#17397=CARTESIAN_POINT ( 'NONE',  ( 54.42435809754115894, 0.4999999999999449329, 6.000000000000136779 ) ) ;
#17404=TOROIDAL_SURFACE ( 'NONE', #5407, 6.500000000000000888, 0.5000000000000000000 ) ;
#17411=EDGE_CURVE ( 'NONE', #19782, #9536, #18455, .T. ) ;
#17436=ADVANCED_FACE ( 'NONE', ( #18346 ), #10917, .T. ) ;
#17451=ADVANCED_FACE ( 'NONE', ( #16675 ), #17404, .T. ) ;
#17466=FACE_OUTER_BOUND ( 'NONE', #6098, .T. ) ;
#17467=LINE ( 'NONE', #21127, #5976 ) ;
#17475=VERTEX_POINT ( 'NONE', #585 ) ;
#17478=EDGE_CURVE ( 'NONE', #10144, #2826, #7750, .T. ) ;
#17497=DIRECTION ( 'NONE',  ( -1.000000000000000000, -2.699383410053119644E-30, -3.330669073875432643E-16 ) ) ;
#17505=CIRCLE ( 'NONE', #10374, 0.5000000000000038858 ) ;
#17506=EDGE_LOOP ( 'NONE', ( #13655, #8008, #16943, #20679 ) ) ;
#17519=LINE ( 'NONE', #23073, #14934 ) ;
#17521=FACE_OUTER_BOUND ( 'NONE', #6474, .T. ) ;
#17542=ADVANCED_FACE ( 'NONE', ( #4447 ), #1369, .T. ) ;
#17564=AXIS2_PLACEMENT_3D ( 'NONE', #22810, #17497, #1288 ) ;
#17565=ORIENTED_EDGE ( 'NONE', *, *, #20002, .T. ) ;
#17585=DIRECTION ( 'NONE',  ( -3.330669073875432643E-16, -4.437342591868153746E-31, 1.000000000000000000 ) ) ;
#17594=DIRECTION ( 'NONE',  ( 0.000000000000000000, -1.000000000000000000, 0.000000000000000000 ) ) ;
#17600=DIRECTION ( 'NONE',  ( -1.000000000000000000, -2.699383410053119644E-30, -3.330669073875432643E-16 ) ) ;
#17606=ORIENTED_EDGE ( 'NONE', *, *, #10575, .F. ) ;
#17611=CARTESIAN_POINT ( 'NONE',  ( 63.53596085922837489, -4.500000000000059508, -6.499999999999957367 ) ) ;
#17613=CIRCLE ( 'NONE', #15740, 0.5000000000000038858 ) ;
#17619=CARTESIAN_POINT ( 'NONE',  ( 110.9706201109471522, -9.453020409440265226, 6.500000000000095923 ) ) ;
#17627=AXIS2_PLACEMENT_3D ( 'NONE', #10907, #113, #11265 ) ;
#17634=EDGE_LOOP ( 'NONE', ( #147, #11813, #20964, #18642 ) ) ;
#17636=PRODUCT_DEFINITION_FORMATION_WITH_SPECIFIED_SOURCE ( 'ANY', '', #7073, .NOT_KNOWN. ) ;
#17640=DIRECTION ( 'NONE',  ( 3.885780586188016830E-16, 4.437342591868156373E-31, -1.000000000000000000 ) ) ;
#17656=ORIENTED_EDGE ( 'NONE', *, *, #22019, .T. ) ;
#17658=VERTEX_POINT ( 'NONE', #12519 ) ;
#17660=DIRECTION ( 'NONE',  ( -1.000000000000000000, -2.699383410053119644E-30, -3.330669073875432643E-16 ) ) ;
#17661=DIRECTION ( 'NONE',  ( -1.000000000000000000, -2.699383410053119644E-30, -3.330669073875432643E-16 ) ) ;
#17667=DIRECTION ( 'NONE',  ( -1.000000000000000000, 4.625929269271439095E-14, -3.854941057726199147E-16 ) ) ;
#17672=PRODUCT_DEFINITION ( 'UNKNOWN', '', #17636, #2995 ) ;
#17682=ORIENTED_EDGE ( 'NONE', *, *, #7805, .F. ) ;
#17686=ORIENTED_EDGE ( 'NONE', *, *, #18864, .T. ) ;
#17694=LINE ( 'NONE', #19708, #8367 ) ;
#17695=LINE ( 'NONE', #7138, #12889 ) ;
#17708=ADVANCED_FACE ( 'NONE', ( #7357 ), #5478, .T. ) ;
#17709=DIRECTION ( 'NONE',  ( 3.330669073875432643E-16, 4.437342591868153746E-31, -1.000000000000000000 ) ) ;
#17723=CYLINDRICAL_SURFACE ( 'NONE', #4204, 0.4999999999999978351 ) ;
#17730=ADVANCED_FACE ( 'NONE', ( #3473 ), #11768, .T. ) ;
#17735=VECTOR ( 'NONE', #2253, 1000.000000000000000 ) ;
#17741=DIRECTION ( 'NONE',  ( -0.6819983600624998088, 0.7313537016191693496, 0.000000000000000000 ) ) ;
#17758=AXIS2_PLACEMENT_3D ( 'NONE', #13268, #693, #2673 ) ;
#17759=LINE ( 'NONE', #3860, #13513 ) ;
#17771=CIRCLE ( 'NONE', #19653, 6.500000000000075495 ) ;
#17778=ORIENTED_EDGE ( 'NONE', *, *, #1118, .F. ) ;
#17789=DIRECTION ( 'NONE',  ( 3.885780586188016830E-16, 4.437342591868156373E-31, -1.000000000000000000 ) ) ;
#17796=CIRCLE ( 'NONE', #20816, 4.500000000000052403 ) ;
#17800=VECTOR ( 'NONE', #601, 1000.000000000000000 ) ;
#17801=AXIS2_PLACEMENT_3D ( 'NONE', #1335, #10492, #4956 ) ;
#17803=DIRECTION ( 'NONE',  ( -3.885780586188016830E-16, -4.437342591868156373E-31, 1.000000000000000000 ) ) ;
#17806=DIRECTION ( 'NONE',  ( 0.6819983600624981435, -0.7313537016191709039, 0.000000000000000000 ) ) ;
#17817=AXIS2_PLACEMENT_3D ( 'NONE', #17850, #12424, #14206 ) ;
#17835=DIRECTION ( 'NONE',  ( -0.7313537016191749007, 0.6819983600624938136, -2.779290820238839172E-15 ) ) ;
#17838=DIRECTION ( 'NONE',  ( 1.000000000000000000, -7.477632011778292156E-48, 3.885780586188017323E-16 ) ) ;
#17843=VERTEX_POINT ( 'NONE', #4154 ) ;
#17846=ORIENTED_EDGE ( 'NONE', *, *, #17270, .F. ) ;
#17850=CARTESIAN_POINT ( 'NONE',  ( 124.5000000000017195, -4.000000000000058620, 1.387778780781445676E-14 ) ) ;
#17861=EDGE_CURVE ( 'NONE', #16898, #10216, #11226, .T. ) ;
#17868=CARTESIAN_POINT ( 'NONE',  ( 109.2950040998454710, -11.69922134891568355, 6.000000000000067502 ) ) ;
#17876=DIRECTION ( 'NONE',  ( -1.000000000000000000, -2.699383410053119644E-30, -3.330669073875432643E-16 ) ) ;
#17877=CARTESIAN_POINT ( 'NONE',  ( 6.500000000000005329, 0.5000000000001669775, 3.469446951953614189E-14 ) ) ;
#17880=CIRCLE ( 'NONE', #12612, 7.000000000000075495 ) ;
#17882=LINE ( 'NONE', #8943, #13435 ) ;
#17888=FACE_OUTER_BOUND ( 'NONE', #19340, .T. ) ;
#17911=CARTESIAN_POINT ( 'NONE',  ( 63.53596085922837489, -2.925414806476733798, -6.499999999999957367 ) ) ;
#17917=CARTESIAN_POINT ( 'NONE',  ( 81.85734743794770907, -6.246200939475199831, 6.000000000000102141 ) ) ;
#17936=PLANE ( 'NONE',  #20474 ) ;
#17940=PLANE ( 'NONE',  #16512 ) ;
#17942=AXIS2_PLACEMENT_3D ( 'NONE', #11680, #16315, #15210 ) ;
#17948=EDGE_CURVE ( 'NONE', #14077, #15916, #16302, .T. ) ;
#17954=FACE_OUTER_BOUND ( 'NONE', #14769, .T. ) ;
#17968=DIRECTION ( 'NONE',  ( 3.885780586187959638E-16, 0.000000000000000000, -1.000000000000000000 ) ) ;
#17988=FACE_OUTER_BOUND ( 'NONE', #20387, .T. ) ;
#17989=ORIENTED_EDGE ( 'NONE', *, *, #20748, .F. ) ;
#17991=ORIENTED_EDGE ( 'NONE', *, *, #17247, .T. ) ;
#17997=VECTOR ( 'NONE', #10875, 1000.000000000000114 ) ;
#18000=EDGE_CURVE ( 'NONE', #7880, #2970, #15546, .T. ) ;
#18016=DIRECTION ( 'NONE',  ( 1.000000000000000000, 4.356083395230605100E-14, 3.854941057726199147E-16 ) ) ;
#18021=VERTEX_POINT ( 'NONE', #19915 ) ;
#18024=EDGE_CURVE ( 'NONE', #2907, #21787, #14062, .T. ) ;
#18031=CARTESIAN_POINT ( 'NONE',  ( 124.5000000000018332, -7.000000000000006217, 6.000000000000088818 ) ) ;
#18043=DIRECTION ( 'NONE',  ( 1.000000000000000000, 2.699383410053119644E-30, 3.330669073875432643E-16 ) ) ;
#18050=EDGE_CURVE ( 'NONE', #21787, #8580, #19796, .T. ) ;
#18059=ORIENTED_EDGE ( 'NONE', *, *, #18823, .T. ) ;
#18070=DIRECTION ( 'NONE',  ( 3.885780586188016830E-16, 4.437342591868156373E-31, -1.000000000000000000 ) ) ;
#18072=EDGE_LOOP ( 'NONE', ( #13788, #10542, #19691, #20447 ) ) ;
#18074=ORIENTED_EDGE ( 'NONE', *, *, #22180, .F. ) ;
#18080=CARTESIAN_POINT ( 'NONE',  ( 83.98338480886823731, -11.64708151429766403, 6.500000000000117240 ) ) ;
#18089=LINE ( 'NONE', #2078, #430 ) ;
#18091=FACE_OUTER_BOUND ( 'NONE', #306, .T. ) ;
#18092=CARTESIAN_POINT ( 'NONE',  ( 77.42435809754134368, -10.99999999999981526, -6.000000000000047073 ) ) ;
#18107=AXIS2_PLACEMENT_3D ( 'NONE', #3012, #22661, #10179 ) ;
#18109=DIRECTION ( 'NONE',  ( 3.032184104443272185E-30, 1.000000000000000000, -7.395570986447005381E-32 ) ) ;
#18126=VECTOR ( 'NONE', #669, 1000.000000000000000 ) ;
#18134=LINE ( 'NONE', #12833, #19279 ) ;
#18145=CIRCLE ( 'NONE', #8016, 6.000000000000063061 ) ;
#18162=ORIENTED_EDGE ( 'NONE', *, *, #9226, .F. ) ;
#18167=TOROIDAL_SURFACE ( 'NONE', #11398, 6.500000000000000888, 0.5000000000000000000 ) ;
#18168=CYLINDRICAL_SURFACE ( 'NONE', #22278, 4.000000000000045297 ) ;
#18180=CARTESIAN_POINT ( 'NONE',  ( 61.48996577904083694, -5.119475911334187224, 6.500000000000130562 ) ) ;
#18184=DIRECTION ( 'NONE',  ( -0.6819983600625061371, -0.7313537016191633544, 0.000000000000000000 ) ) ;
#18185=DIRECTION ( 'NONE',  ( 0.000000000000000000, 0.000000000000000000, 1.000000000000000000 ) ) ;
#18188=AXIS2_PLACEMENT_3D ( 'NONE', #2336, #21993, #9520 ) ;
#18192=AXIS2_PLACEMENT_3D ( 'NONE', #10318, #8559, #17968 ) ;
#18193=EDGE_CURVE ( 'NONE', #6496, #5349, #2419, .T. ) ;
#18194=ORIENTED_EDGE ( 'NONE', *, *, #17314, .T. ) ;
#18195=DIRECTION ( 'NONE',  ( -3.330669073875432643E-16, -4.437342591868153746E-31, 1.000000000000000000 ) ) ;
#18202=DIRECTION ( 'NONE',  ( -1.000000000000000000, 5.055479844275211845E-14, -3.717264591378832268E-16 ) ) ;
#18211=CARTESIAN_POINT ( 'NONE',  ( 54.42435809754108078, -4.000000000000003553, 6.500000000000081712 ) ) ;
#18219=EDGE_LOOP ( 'NONE', ( #2728, #7804, #5163, #6299 ) ) ;
#18235=CYLINDRICAL_SURFACE ( 'NONE', #4030, 0.5000000000000038858 ) ;
#18248=CARTESIAN_POINT ( 'NONE',  ( 66.26395429947837101, -4.000000000000003553, 6.500000000000110134 ) ) ;
#18252=DIRECTION ( 'NONE',  ( -0.6819983600625060260, -0.7313537016191635765, -6.106365041599011361E-16 ) ) ;
#18255=CARTESIAN_POINT ( 'NONE',  ( 124.5000000000019469, -13.52760560296373171, -6.938893903907228378E-15 ) ) ;
#18261=DIRECTION ( 'NONE',  ( -1.000000000000000000, -2.699383410053119644E-30, -3.330669073875432643E-16 ) ) ;
#18263=DIRECTION ( 'NONE',  ( 1.000000000000000000, -7.477632011778292156E-48, 3.885780586188017323E-16 ) ) ;
#18270=ORIENTED_EDGE ( 'NONE', *, *, #13956, .F. ) ;
#18271=VERTEX_POINT ( 'NONE', #11530 ) ;
#18273=VECTOR ( 'NONE', #2891, 1000.000000000000000 ) ;
#18275=CARTESIAN_POINT ( 'NONE',  ( 59.19834661797866460, 1.119475911334100182, 6.500000000000130562 ) ) ;
#18277=VERTEX_POINT ( 'NONE', #11421 ) ;
#18293=EDGE_CURVE ( 'NONE', #8517, #21954, #9563, .T. ) ;
#18295=VECTOR ( 'NONE', #16608, 1000.000000000000000 ) ;
#18296=CARTESIAN_POINT ( 'NONE',  ( 77.42435809754141474, -6.499999999999811706, 6.000000000000095923 ) ) ;
#18304=AXIS2_PLACEMENT_3D ( 'NONE', #16930, #21162, #6371 ) ;
#18306=EDGE_LOOP ( 'NONE', ( #271, #13672, #19346, #10860 ) ) ;
#18308=VECTOR ( 'NONE', #15736, 1000.000000000000000 ) ;
#18310=CARTESIAN_POINT ( 'NONE',  ( 88.75737332930583534, -11.02760560296348125, -6.500000000000047073 ) ) ;
#18335=AXIS2_PLACEMENT_3D ( 'NONE', #8330, #2922, #1391 ) ;
#18341=AXIS2_PLACEMENT_3D ( 'NONE', #22843, #13893, #3201 ) ;
#18342=CARTESIAN_POINT ( 'NONE',  ( 73.50000000000116529, -13.52760560296348302, 3.469446951953614189E-14 ) ) ;
#18343=AXIS2_PLACEMENT_3D ( 'NONE', #5539, #9181, #14005 ) ;
#18346=FACE_OUTER_BOUND ( 'NONE', #19545, .T. ) ;
#18348=CARTESIAN_POINT ( 'NONE',  ( 124.5000000000019185, -7.000000000000062172, -5.999999999999984901 ) ) ;
#18351=CYLINDRICAL_SURFACE ( 'NONE', #13475, 0.4999999999999978351 ) ;
#18358=SHAPE_DEFINITION_REPRESENTATION ( #1609, #15574 ) ;
#18360=ORIENTED_EDGE ( 'NONE', *, *, #4321, .F. ) ;
#18361=EDGE_CURVE ( 'NONE', #4169, #4164, #13545, .T. ) ;
#18376=FACE_OUTER_BOUND ( 'NONE', #6414, .T. ) ;
#18378=CARTESIAN_POINT ( 'NONE',  ( 77.42435809754137210, -6.999999999999811706, 6.500000000000081712 ) ) ;
#18393=DIRECTION ( 'NONE',  ( -0.6819983600624981435, -0.7313537016191709039, 0.000000000000000000 ) ) ;
#18403=DIRECTION ( 'NONE',  ( -3.885780586188016830E-16, -4.437342591868156373E-31, 1.000000000000000000 ) ) ;
#18416=EDGE_CURVE ( 'NONE', #18645, #15578, #17384, .T. ) ;
#18422=CARTESIAN_POINT ( 'NONE',  ( 66.26395429947839943, 0.000000000000000000, 6.000000000000178524 ) ) ;
#18427=PLANE ( 'NONE',  #8334 ) ;
#18444=ORIENTED_EDGE ( 'NONE', *, *, #3922, .T. ) ;
#18445=CARTESIAN_POINT ( 'NONE',  ( 112.6756160111034575, -11.28140466348828674, -6.500000000000040856 ) ) ;
#18452=DIRECTION ( 'NONE',  ( -3.885780586188016830E-16, -4.437342591868156373E-31, 1.000000000000000000 ) ) ;
#18453=CARTESIAN_POINT ( 'NONE',  ( 86.02937988905580369, -9.453020409440155092, -6.499999999999943157 ) ) ;
#18454=CARTESIAN_POINT ( 'NONE',  ( 2.498001805406602216E-13, 3.000000000000002665, 6.500000000000103029 ) ) ;
#18455=LINE ( 'NONE', #2226, #10647 ) ;
#18461=LINE ( 'NONE', #16452, #5958 ) ;
#18470=AXIS2_PLACEMENT_3D ( 'NONE', #11830, #21011, #8537 ) ;
#18480=DIRECTION ( 'NONE',  ( 3.032184104443272185E-30, 1.000000000000000000, -7.395570986447005381E-32 ) ) ;
#18504=FACE_OUTER_BOUND ( 'NONE', #21475, .T. ) ;
#18507=DIRECTION ( 'NONE',  ( 3.885780586188016830E-16, 4.437342591868156373E-31, -1.000000000000000000 ) ) ;
#18524=AXIS2_PLACEMENT_3D ( 'NONE', #12243, #16236, #10497 ) ;
#18538=DIRECTION ( 'NONE',  ( 1.000000000000000000, 2.699383410053119293E-30, 4.336808689941968432E-16 ) ) ;
#18539=AXIS2_PLACEMENT_3D ( 'NONE', #1060, #20582, #22700 ) ;
#18550=DIRECTION ( 'NONE',  ( 0.000000000000000000, 0.000000000000000000, 1.000000000000000000 ) ) ;
#18563=CARTESIAN_POINT ( 'NONE',  ( 119.5756419024615269, -4.500000000000003553, 6.500000000000123457 ) ) ;
#18564=EDGE_LOOP ( 'NONE', ( #7569, #16152, #19544, #11485 ) ) ;
#18573=ADVANCED_FACE ( 'NONE', ( #9523 ), #2230, .F. ) ;
#18592=ORIENTED_EDGE ( 'NONE', *, *, #22639, .F. ) ;
#18608=( NAMED_UNIT ( * ) PLANE_ANGLE_UNIT ( ) SI_UNIT ( $, .RADIAN. ) );
#18614=ORIENTED_EDGE ( 'NONE', *, *, #6786, .T. ) ;
#18623=CARTESIAN_POINT ( 'NONE',  ( 119.5756419024615269, -4.000000000000003553, 6.500000000000123457 ) ) ;
#18625=ORIENTED_EDGE ( 'NONE', *, *, #17222, .F. ) ;
#18642=ORIENTED_EDGE ( 'NONE', *, *, #22120, .F. ) ;
#18644=VERTEX_POINT ( 'NONE', #467 ) ;
#18645=VERTEX_POINT ( 'NONE', #16680 ) ;
#18651=VERTEX_POINT ( 'NONE', #7530 ) ;
#18655=DIRECTION ( 'NONE',  ( -0.7313537016191731244, 0.6819983600624957010, -5.924440990721420203E-17 ) ) ;
#18661=AXIS2_PLACEMENT_3D ( 'NONE', #19337, #1453, #19446 ) ;
#18675=CARTESIAN_POINT ( 'NONE',  ( 6.500000000000227374, 1.665334536937734811E-13, 6.000000000000213163 ) ) ;
#18678=DIRECTION ( 'NONE',  ( -1.000000000000000000, 0.000000000000000000, -4.336808689941968432E-16 ) ) ;
#18698=ORIENTED_EDGE ( 'NONE', *, *, #18361, .F. ) ;
#18701=CIRCLE ( 'NONE', #1814, 4.500000000000045297 ) ;
#18714=DIRECTION ( 'NONE',  ( 0.7313537016191731244, -0.6819983600624958120, 5.924440990721420203E-17 ) ) ;
#18716=( NAMED_UNIT ( * ) SI_UNIT ( $, .STERADIAN. ) SOLID_ANGLE_UNIT ( ) );
#18717=ADVANCED_FACE ( 'NONE', ( #19048 ), #9994, .T. ) ;
#18732=ORIENTED_EDGE ( 'NONE', *, *, #18766, .F. ) ;
#18734=ORIENTED_EDGE ( 'NONE', *, *, #18823, .F. ) ;
#18747=EDGE_CURVE ( 'NONE', #11343, #5312, #2817, .T. ) ;
#18748=EDGE_CURVE ( 'NONE', #10144, #17843, #21563, .T. ) ;
#18766=EDGE_CURVE ( 'NONE', #14732, #273, #8106, .T. ) ;
#18769=VECTOR ( 'NONE', #8475, 1000.000000000000114 ) ;
#18776=DIRECTION ( 'NONE',  ( -1.000000000000000000, -5.598259082250514647E-17, -3.330669073875432643E-16 ) ) ;
#18780=DIRECTION ( 'NONE',  ( 3.032184104443272185E-30, 1.000000000000000000, -7.395570986447005381E-32 ) ) ;
#18790=DIRECTION ( 'NONE',  ( 0.6819983600625072473, 0.7313537016191623552, 0.000000000000000000 ) ) ;
#18795=ORIENTED_EDGE ( 'NONE', *, *, #13244, .T. ) ;
#18796=ORIENTED_EDGE ( 'NONE', *, *, #18766, .T. ) ;
#18817=ORIENTED_EDGE ( 'NONE', *, *, #12988, .T. ) ;
#18823=EDGE_CURVE ( 'NONE', #16867, #4929, #7166, .T. ) ;
#18825=EDGE_LOOP ( 'NONE', ( #9096, #2178, #18625, #3847 ) ) ;
#18840=TOROIDAL_SURFACE ( 'NONE', #18107, 6.500000000000000888, 0.5000000000000000000 ) ;
#18843=VERTEX_POINT ( 'NONE', #19383 ) ;
#18846=ORIENTED_EDGE ( 'NONE', *, *, #5954, .T. ) ;
#18852=FACE_OUTER_BOUND ( 'NONE', #22794, .T. ) ;
#18853=DIRECTION ( 'NONE',  ( 1.000000000000000000, 2.699383410053119644E-30, 3.330669073875432643E-16 ) ) ;
#18859=CIRCLE ( 'NONE', #21871, 7.000000000000075495 ) ;
#18864=EDGE_CURVE ( 'NONE', #11435, #2970, #14219, .T. ) ;
#18885=ORIENTED_EDGE ( 'NONE', *, *, #22769, .F. ) ;
#18891=DIRECTION ( 'NONE',  ( -1.000000000000000000, -2.699383410053119644E-30, -3.330669073875432643E-16 ) ) ;
#18921=CIRCLE ( 'NONE', #8416, 7.000000000000075495 ) ;
#18940=TOROIDAL_SURFACE ( 'NONE', #2389, 6.500000000000000888, 0.5000000000000000000 ) ;
#18943=ORIENTED_EDGE ( 'NONE', *, *, #8855, .T. ) ;
#18945=CARTESIAN_POINT ( 'NONE',  ( 82.19834661797897013, -4.499999999999809930, 6.500000000000151879 ) ) ;
#18948=VECTOR ( 'NONE', #4508, 1000.000000000000000 ) ;
#18953=CIRCLE ( 'NONE', #23098, 6.500000000000075495 ) ;
#18964=ORIENTED_EDGE ( 'NONE', *, *, #12081, .F. ) ;
#18973=ORIENTED_EDGE ( 'NONE', *, *, #4507, .F. ) ;
#18978=CARTESIAN_POINT ( 'NONE',  ( 113.0166151911346759, -11.64708151429785765, -6.500000000000040856 ) ) ;
#18983=AXIS2_PLACEMENT_3D ( 'NONE', #17619, #21516, #8803 ) ;
#18987=DIRECTION ( 'NONE',  ( -3.330669073875432643E-16, -4.437342591868153746E-31, 1.000000000000000000 ) ) ;
#18988=DIRECTION ( 'NONE',  ( -0.6819983600624976994, -0.7313537016191713480, 0.000000000000000000 ) ) ;
#18992=LINE ( 'NONE', #11683, #15316 ) ;
#18995=EDGE_CURVE ( 'NONE', #16118, #8988, #6525, .T. ) ;
#18996=ORIENTED_EDGE ( 'NONE', *, *, #22779, .T. ) ;
#19017=ADVANCED_FACE ( 'NONE', ( #18091 ), #15012, .T. ) ;
#19023=ORIENTED_EDGE ( 'NONE', *, *, #2640, .F. ) ;
#19030=ORIENTED_EDGE ( 'NONE', *, *, #10810, .F. ) ;
#19037=DIRECTION ( 'NONE',  ( 1.000000000000000000, 5.501551595240671658E-14, 3.717264591378832268E-16 ) ) ;
#19039=CIRCLE ( 'NONE', #14149, 0.4999999999999984457 ) ;
#19040=DIRECTION ( 'NONE',  ( 0.000000000000000000, 0.000000000000000000, 1.000000000000000000 ) ) ;
#19048=FACE_OUTER_BOUND ( 'NONE', #20450, .T. ) ;
#19050=DIRECTION ( 'NONE',  ( -1.000000000000000000, -2.699383410053119644E-30, -3.330669073875432643E-16 ) ) ;
#19057=DIRECTION ( 'NONE',  ( 1.000000000000000000, 2.699383410053119644E-30, 3.330669073875432643E-16 ) ) ;
#19078=ORIENTED_EDGE ( 'NONE', *, *, #16080, .T. ) ;
#19082=EDGE_LOOP ( 'NONE', ( #15794, #19576, #3880, #20050 ) ) ;
#19087=DIRECTION ( 'NONE',  ( 0.000000000000000000, 0.000000000000000000, 1.000000000000000000 ) ) ;
#19089=DIRECTION ( 'NONE',  ( -3.885780586188016830E-16, -4.437342591868156373E-31, 1.000000000000000000 ) ) ;
#19128=DIRECTION ( 'NONE',  ( -1.000000000000000000, -2.699383410053119644E-30, -3.330669073875432643E-16 ) ) ;
#19149=AXIS2_PLACEMENT_3D ( 'NONE', #4762, #11931, #18891 ) ;
#19157=CARTESIAN_POINT ( 'NONE',  ( 77.42435809754135789, -6.499999999999811706, 6.500000000000137668 ) ) ;
#19158=DIRECTION ( 'NONE',  ( -1.000000000000000000, 0.000000000000000000, -3.330669073875427220E-16 ) ) ;
#19168=EDGE_CURVE ( 'NONE', #14827, #18651, #11409, .T. ) ;
#19171=DIRECTION ( 'NONE',  ( -1.000000000000000000, -5.598259082250514647E-17, -3.330669073875432643E-16 ) ) ;
#19177=EDGE_CURVE ( 'NONE', #7460, #23117, #12149, .T. ) ;
#19190=ORIENTED_EDGE ( 'NONE', *, *, #16958, .T. ) ;
#19193=ORIENTED_EDGE ( 'NONE', *, *, #15551, .F. ) ;
#19195=ORIENTED_EDGE ( 'NONE', *, *, #23074, .F. ) ;
#19212=AXIS2_PLACEMENT_3D ( 'NONE', #14445, #3619, #21627 ) ;
#19230=DIRECTION ( 'NONE',  ( -1.000000000000000000, 4.981134552447635210E-14, -3.717264591378832268E-16 ) ) ;
#19247=ADVANCED_FACE ( 'NONE', ( #6434 ), #12543, .T. ) ;
#19254=CARTESIAN_POINT ( 'NONE',  ( 63.82609305959173440, -6.614286113036355275, 6.000000000000095923 ) ) ;
#19275=AXIS2_PLACEMENT_3D ( 'NONE', #1983, #12580, #10811 ) ;
#19276=CIRCLE ( 'NONE', #5005, 4.000000000000045297 ) ;
#19279=VECTOR ( 'NONE', #9426, 1000.000000000000000 ) ;
#19284=DIRECTION ( 'NONE',  ( 0.000000000000000000, 0.000000000000000000, 1.000000000000000000 ) ) ;
#19292=DIRECTION ( 'NONE',  ( 0.7313537016191730133, -0.6819983600624958120, 5.924440990721418971E-17 ) ) ;
#19297=VECTOR ( 'NONE', #15493, 1000.000000000000000 ) ;
#19302=VECTOR ( 'NONE', #20011, 1000.000000000000000 ) ;
#19329=CARTESIAN_POINT ( 'NONE',  ( 77.42435809754141474, -4.499999999999809930, 6.000000000000095923 ) ) ;
#19333=EDGE_CURVE ( 'NONE', #8988, #4062, #19692, .T. ) ;
#19337=CARTESIAN_POINT ( 'NONE',  ( 77.42435809754135789, -10.99999999999981526, 6.500000000000123457 ) ) ;
#19340=EDGE_LOOP ( 'NONE', ( #15016, #6631, #11573, #1918 ) ) ;
#19346=ORIENTED_EDGE ( 'NONE', *, *, #7716, .F. ) ;
#19348=VECTOR ( 'NONE', #941, 1000.000000000000000 ) ;
#19351=DIRECTION ( 'NONE',  ( -5.598259082250514647E-17, 1.000000000000000000, -6.162975822039315660E-32 ) ) ;
#19365=CARTESIAN_POINT ( 'NONE',  ( 108.2426266706971205, -11.02760560296367487, -6.500000000000075495 ) ) ;
#19367=VERTEX_POINT ( 'NONE', #14525 ) ;
#19369=ORIENTED_EDGE ( 'NONE', *, *, #12117, .F. ) ;
#19370=ADVANCED_FACE ( 'NONE', ( #9665 ), #22309, .T. ) ;
#19377=CARTESIAN_POINT ( 'NONE',  ( 80.15235153779141797, -8.074585193523137860, -6.500000000000019540 ) ) ;
#19383=CARTESIAN_POINT ( 'NONE',  ( 54.42435809754109499, 0.4999999999999449329, 6.500000000000144773 ) ) ;
#19387=CARTESIAN_POINT ( 'NONE',  ( 54.42435809754106657, -4.000000000000003553, 6.000000000000136779 ) ) ;
#19396=CARTESIAN_POINT ( 'NONE',  ( 73.50000000000116529, -3.999999999999809042, -2.549999999999874589 ) ) ;
#19401=ORIENTED_EDGE ( 'NONE', *, *, #21922, .F. ) ;
#19404=CYLINDRICAL_SURFACE ( 'NONE', #1053, 0.5000000000000038858 ) ;
#19423=EDGE_LOOP ( 'NONE', ( #2265, #5342, #22326, #2142 ) ) ;
#19426=CARTESIAN_POINT ( 'NONE',  ( 66.26395429947837101, 0.000000000000000000, -5.999999999999908518 ) ) ;
#19428=CYLINDRICAL_SURFACE ( 'NONE', #14702, 0.5000000000000038858 ) ;
#19446=DIRECTION ( 'NONE',  ( 1.000000000000000000, 4.780126911580487002E-14, 3.854941057726199147E-16 ) ) ;
#19452=ORIENTED_EDGE ( 'NONE', *, *, #5944, .F. ) ;
#19453=CIRCLE ( 'NONE', #16433, 4.000000000000045297 ) ;
#19473=EDGE_CURVE ( 'NONE', #21954, #6421, #10153, .T. ) ;
#19476=DIRECTION ( 'NONE',  ( 0.000000000000000000, 0.000000000000000000, -1.000000000000000000 ) ) ;
#19484=PLANE ( 'NONE',  #2595 ) ;
#19485=CIRCLE ( 'NONE', #1091, 4.000000000000045297 ) ;
#19486=CARTESIAN_POINT ( 'NONE',  ( 81.04599508018866061, -4.805938895142331191, -5.999999999999950262 ) ) ;
#19489=ORIENTED_EDGE ( 'NONE', *, *, #2965, .F. ) ;
#19501=AXIS2_PLACEMENT_3D ( 'NONE', #22075, #13140, #14543 ) ;
#19544=ORIENTED_EDGE ( 'NONE', *, *, #5954, .F. ) ;
#19545=EDGE_LOOP ( 'NONE', ( #22411, #8667, #22058, #13732 ) ) ;
#19546=ORIENTED_EDGE ( 'NONE', *, *, #7849, .F. ) ;
#19565=VERTEX_POINT ( 'NONE', #3223 ) ;
#19566=ADVANCED_FACE ( 'NONE', ( #20872 ), #20754, .F. ) ;
#19576=ORIENTED_EDGE ( 'NONE', *, *, #22769, .T. ) ;
#19586=VECTOR ( 'NONE', #21015, 1000.000000000000114 ) ;
#19593=EDGE_LOOP ( 'NONE', ( #14800, #9712, #4842, #6391 ) ) ;
#19607=CARTESIAN_POINT ( 'NONE',  ( 124.5000000000018900, -6.500000000000061284, -6.500000000000040856 ) ) ;
#19634=CARTESIAN_POINT ( 'NONE',  ( 119.5756419024615269, -4.500000000000003553, 6.500000000000123457 ) ) ;
#19651=FACE_OUTER_BOUND ( 'NONE', #8090, .T. ) ;
#19653=AXIS2_PLACEMENT_3D ( 'NONE', #4766, #22897, #13604 ) ;
#19656=CIRCLE ( 'NONE', #20023, 0.5000000000000038858 ) ;
#19671=AXIS2_PLACEMENT_3D ( 'NONE', #21746, #677, #18550 ) ;
#19683=CARTESIAN_POINT ( 'NONE',  ( 114.8016533820240852, -5.880524088665878502, -5.999999999999928946 ) ) ;
#19688=PLANE ( 'NONE',  #5175 ) ;
#19691=ORIENTED_EDGE ( 'NONE', *, *, #1110, .F. ) ;
#19692=CIRCLE ( 'NONE', #2405, 0.5000000000000038858 ) ;
#19707=CARTESIAN_POINT ( 'NONE',  ( 113.0166151911346759, -11.64708151429785765, -6.500000000000040856 ) ) ;
#19708=CARTESIAN_POINT ( 'NONE',  ( 86.02937988905580369, -9.453020409440155092, 6.500000000000165201 ) ) ;
#19724=EDGE_LOOP ( 'NONE', ( #9945, #8027, #314, #18162 ) ) ;
#19726=PLANE ( 'NONE',  #730 ) ;
#19728=VERTEX_POINT ( 'NONE', #12607 ) ;
#19733=DIRECTION ( 'NONE',  ( -0.7313537016191730133, 0.6819983600624959230, -5.924440990721418971E-17 ) ) ;
#19735=CARTESIAN_POINT ( 'NONE',  ( 73.50000000000115108, -6.999999999999811706, -6.938893903907228378E-15 ) ) ;
#19743=EDGE_CURVE ( 'NONE', #16151, #13355, #3187, .T. ) ;
#19751=DIRECTION ( 'NONE',  ( -1.000000000000000000, -2.699383410053119644E-30, -3.330669073875432643E-16 ) ) ;
#19774=ADVANCED_FACE ( 'NONE', ( #18376 ), #5901, .T. ) ;
#19782=VERTEX_POINT ( 'NONE', #11299 ) ;
#19796=LINE ( 'NONE', #23108, #6178 ) ;
#19801=FACE_OUTER_BOUND ( 'NONE', #10456, .T. ) ;
#19804=ADVANCED_FACE ( 'NONE', ( #5800 ), #12961, .T. ) ;
#19806=ORIENTED_EDGE ( 'NONE', *, *, #4175, .F. ) ;
#19809=ORIENTED_EDGE ( 'NONE', *, *, #14851, .T. ) ;
#19818=CARTESIAN_POINT ( 'NONE',  ( 58.85734743794746038, 0.7537990605245292741, 6.500000000000123457 ) ) ;
#19834=EDGE_LOOP ( 'NONE', ( #7262, #2215, #19030, #8841 ) ) ;
#19837=VECTOR ( 'NONE', #7336, 1000.000000000000000 ) ;
#19840=ORIENTED_EDGE ( 'NONE', *, *, #5927, .T. ) ;
#19842=CARTESIAN_POINT ( 'NONE',  ( 88.75737332930587797, -11.02760560296348125, 6.500000000000075495 ) ) ;
#19851=DIRECTION ( 'NONE',  ( 3.885780586188016830E-16, 4.437342591868156373E-31, -1.000000000000000000 ) ) ;
#19856=CIRCLE ( 'NONE', #330, 4.500000000000045297 ) ;
#19862=VERTEX_POINT ( 'NONE', #17169 ) ;
#19869=DIRECTION ( 'NONE',  ( -0.7313537016191735685, 0.6819983600624951459, -3.923113172947598083E-16 ) ) ;
#19909=LINE ( 'NONE', #17911, #12781 ) ;
#19914=AXIS2_PLACEMENT_3D ( 'NONE', #14866, #9459, #5474 ) ;
#19915=CARTESIAN_POINT ( 'NONE',  ( 54.42435809754115894, -8.326672684688674053E-14, -5.999999999999950262 ) ) ;
#19938=CARTESIAN_POINT ( 'NONE',  ( 110.9706201109471522, -11.02760560296359138, 6.500000000000095923 ) ) ;
#19957=FACE_OUTER_BOUND ( 'NONE', #5200, .T. ) ;
#20002=EDGE_CURVE ( 'NONE', #19565, #11343, #5059, .T. ) ;
#20009=ORIENTED_EDGE ( 'NONE', *, *, #7529, .T. ) ;
#20011=DIRECTION ( 'NONE',  ( -3.241725282392603095E-30, -1.000000000000000000, 2.218671295934100958E-31 ) ) ;
#20021=DIRECTION ( 'NONE',  ( 1.000000000000000000, 0.000000000000000000, 4.336808689941968432E-16 ) ) ;
#20023=AXIS2_PLACEMENT_3D ( 'NONE', #15406, #22593, #8480 ) ;
#20030=DIRECTION ( 'NONE',  ( -1.000000000000000000, -5.598259082250514647E-17, -3.330669073875432643E-16 ) ) ;
#20050=ORIENTED_EDGE ( 'NONE', *, *, #22639, .T. ) ;
#20051=AXIS2_PLACEMENT_3D ( 'NONE', #5206, #4733, #23214 ) ;
#20070=EDGE_LOOP ( 'NONE', ( #6529, #19369 ) ) ;
#20077=CARTESIAN_POINT ( 'NONE',  ( 88.75737332930593482, -6.527605602963476805, -6.499999999999929834 ) ) ;
#20100=ORIENTED_EDGE ( 'NONE', *, *, #1110, .T. ) ;
#20110=CARTESIAN_POINT ( 'NONE',  ( 77.42435809754134368, -10.99999999999981526, -6.000000000000047073 ) ) ;
#20116=DIRECTION ( 'NONE',  ( 1.000000000000000000, 2.699383410053119644E-30, 3.330669073875432643E-16 ) ) ;
#20120=TOROIDAL_SURFACE ( 'NONE', #3960, 6.000000000000000000, 0.5000000000000000000 ) ;
#20133=DIRECTION ( 'NONE',  ( -1.000000000000000000, 0.000000000000000000, -4.336808689941968432E-16 ) ) ;
#20135=DIRECTION ( 'NONE',  ( -0.7313537016191730133, 0.6819983600624958120, -5.924440990721418971E-17 ) ) ;
#20159=ORIENTED_EDGE ( 'NONE', *, *, #17270, .T. ) ;
#20163=EDGE_LOOP ( 'NONE', ( #1160, #11026, #19023, #16436 ) ) ;
#20178=VERTEX_POINT ( 'NONE', #12811 ) ;
#20186=VECTOR ( 'NONE', #4357, 1000.000000000000000 ) ;
#20201=EDGE_CURVE ( 'NONE', #11516, #14827, #2925, .T. ) ;
#20207=CIRCLE ( 'NONE', #10054, 4.000000000000045297 ) ;
#20214=DIRECTION ( 'NONE',  ( 0.000000000000000000, 0.000000000000000000, 1.000000000000000000 ) ) ;
#20220=FACE_OUTER_BOUND ( 'NONE', #2643, .T. ) ;
#20225=LINE ( 'NONE', #18445, #6532 ) ;
#20231=DIRECTION ( 'NONE',  ( 0.7313537016191730133, -0.6819983600624959230, 5.924440990721418971E-17 ) ) ;
#20242=VECTOR ( 'NONE', #20374, 1000.000000000000000 ) ;
#20266=LINE ( 'NONE', #4128, #12652 ) ;
#20284=CARTESIAN_POINT ( 'NONE',  ( 119.5756419024615838, -6.500000000000005329, 6.000000000000158096 ) ) ;
#20297=ADVANCED_FACE ( 'NONE', ( #2684 ), #23126, .T. ) ;
#20330=EDGE_CURVE ( 'NONE', #4062, #8320, #20871, .T. ) ;
#20355=CIRCLE ( 'NONE', #1566, 0.4999999999999978351 ) ;
#20370=ADVANCED_FACE ( 'NONE', ( #6689 ), #3508, .T. ) ;
#20374=DIRECTION ( 'NONE',  ( -0.7313537016191746787, -0.6819983600624940356, -1.072890437865584409E-16 ) ) ;
#20376=CIRCLE ( 'NONE', #6490, 4.000000000000045297 ) ;
#20387=EDGE_LOOP ( 'NONE', ( #13931, #16866, #19190, #18059 ) ) ;
#20390=ORIENTED_EDGE ( 'NONE', *, *, #8652, .T. ) ;
#20392=DIRECTION ( 'NONE',  ( -1.000000000000000000, -2.699383410053119644E-30, -3.330669073875432643E-16 ) ) ;
#20399=CIRCLE ( 'NONE', #22649, 7.000000000000075495 ) ;
#20402=VECTOR ( 'NONE', #14739, 1000.000000000000000 ) ;
#20403=CARTESIAN_POINT ( 'NONE',  ( 54.42435809754109499, 2.499999999999946709, 6.500000000000144773 ) ) ;
#20408=DIRECTION ( 'NONE',  ( -3.330669073875432643E-16, -4.437342591868153746E-31, 1.000000000000000000 ) ) ;
#20418=CIRCLE ( 'NONE', #9148, 4.500000000000052403 ) ;
#20431=AXIS2_PLACEMENT_3D ( 'NONE', #12170, #17585, #22457 ) ;
#20439=EDGE_CURVE ( 'NONE', #6969, #9218, #12555, .T. ) ;
#20440=DIRECTION ( 'NONE',  ( -1.000000000000000000, -2.699383410053119644E-30, -3.330669073875432643E-16 ) ) ;
#20441=DIRECTION ( 'NONE',  ( 3.032184104443272185E-30, 1.000000000000000000, -7.395570986447005381E-32 ) ) ;
#20447=ORIENTED_EDGE ( 'NONE', *, *, #20002, .F. ) ;
#20450=EDGE_LOOP ( 'NONE', ( #16749, #5383, #4705, #4629 ) ) ;
#20451=CIRCLE ( 'NONE', #12172, 0.4999999999999990563 ) ;
#20461=DIRECTION ( 'NONE',  ( -1.000000000000000000, 5.319818659662146787E-14, -3.854941057726193231E-16 ) ) ;
#20462=DIRECTION ( 'NONE',  ( -1.000000000000000000, -2.699383410053119644E-30, -3.330669073875432643E-16 ) ) ;
#20473=DIRECTION ( 'NONE',  ( 1.000000000000000000, 2.699383410053119644E-30, 3.330669073875432643E-16 ) ) ;
#20474=AXIS2_PLACEMENT_3D ( 'NONE', #9000, #14633, #1920 ) ;
#20482=EDGE_CURVE ( 'NONE', #2970, #11432, #5973, .T. ) ;
#20490=ADVANCED_FACE ( 'NONE', ( #14549 ), #2197, .T. ) ;
#20500=CARTESIAN_POINT ( 'NONE',  ( 81.85734743794770907, -6.246200939475254899, -6.499999999999970690 ) ) ;
#20503=CARTESIAN_POINT ( 'NONE',  ( 66.26395429947832838, -7.000000000000006217, 6.000000000000172307 ) ) ;
#20514=ORIENTED_EDGE ( 'NONE', *, *, #7206, .T. ) ;
#20529=DIRECTION ( 'NONE',  ( 3.885780586188016830E-16, 4.437342591868156373E-31, -1.000000000000000000 ) ) ;
#20530=DIRECTION ( 'NONE',  ( 1.000000000000000000, 2.699383410053119644E-30, 3.330669073875432643E-16 ) ) ;
#20552=AXIS2_PLACEMENT_3D ( 'NONE', #15254, #4791, #19037 ) ;
#20562=ORIENTED_EDGE ( 'NONE', *, *, #5085, .T. ) ;
#20582=DIRECTION ( 'NONE',  ( -1.000000000000000000, -2.699383410053119644E-30, -3.330669073875432643E-16 ) ) ;
#20586=EDGE_CURVE ( 'NONE', #3634, #11343, #7384, .T. ) ;
#20587=CARTESIAN_POINT ( 'NONE',  ( 88.75737332930587797, -10.52760560296347947, -6.000000000000067502 ) ) ;
#20596=EDGE_CURVE ( 'NONE', #16591, #20921, #18089, .T. ) ;
#20603=DIRECTION ( 'NONE',  ( 3.885780586187836378E-16, 0.000000000000000000, -1.000000000000000000 ) ) ;
#20611=DIRECTION ( 'NONE',  ( 1.000000000000000000, 0.000000000000000000, 2.668805347656595124E-16 ) ) ;
#20628=EDGE_CURVE ( 'NONE', #15636, #4169, #1549, .T. ) ;
#20630=ADVANCED_FACE ( 'NONE', ( #7843 ), #21841, .T. ) ;
#20646=CARTESIAN_POINT ( 'NONE',  ( 116.8476484622116232, -8.074585193523331483, 6.500000000000040856 ) ) ;
#20654=ORIENTED_EDGE ( 'NONE', *, *, #20586, .T. ) ;
#20679=ORIENTED_EDGE ( 'NONE', *, *, #22725, .F. ) ;
#20694=CARTESIAN_POINT ( 'NONE',  ( 54.42435809754109499, 2.999999999999947153, 6.500000000000144773 ) ) ;
#20734=ORIENTED_EDGE ( 'NONE', *, *, #6967, .T. ) ;
#20742=EDGE_LOOP ( 'NONE', ( #8313, #19840, #4459, #1518 ) ) ;
#20745=FACE_OUTER_BOUND ( 'NONE', #374, .T. ) ;
#20746=ADVANCED_FACE ( 'NONE', ( #15700 ), #22899, .T. ) ;
#20747=LINE ( 'NONE', #21091, #15534 ) ;
#20748=EDGE_CURVE ( 'NONE', #6130, #15653, #12284, .T. ) ;
#20754=CYLINDRICAL_SURFACE ( 'NONE', #13697, 4.000000000000045297 ) ;
#20757=CIRCLE ( 'NONE', #1578, 4.000000000000045297 ) ;
#20758=AXIS2_PLACEMENT_3D ( 'NONE', #1614, #1949, #9140 ) ;
#20765=DIRECTION ( 'NONE',  ( 3.885780586188016830E-16, 4.437342591868156373E-31, -1.000000000000000000 ) ) ;
#20772=ORIENTED_EDGE ( 'NONE', *, *, #22021, .T. ) ;
#20773=ORIENTED_EDGE ( 'NONE', *, *, #8562, .F. ) ;
#20779=EDGE_CURVE ( 'NONE', #19367, #12208, #5316, .T. ) ;
#20799=LINE ( 'NONE', #11711, #11892 ) ;
#20800=VECTOR ( 'NONE', #5801, 1000.000000000000114 ) ;
#20812=VECTOR ( 'NONE', #3046, 1000.000000000000000 ) ;
#20816=AXIS2_PLACEMENT_3D ( 'NONE', #11273, #457, #20461 ) ;
#20822=DIRECTION ( 'NONE',  ( -1.000000000000000000, -2.699383410053119644E-30, -3.330669073875432643E-16 ) ) ;
#20836=MANIFOLD_SOLID_BREP ( 'Fillet1', #552 ) ;
#20838=ORIENTED_EDGE ( 'NONE', *, *, #766, .F. ) ;
#20855=DIRECTION ( 'NONE',  ( 0.6819983600624998088, 0.7313537016191693496, 0.000000000000000000 ) ) ;
#20860=VERTEX_POINT ( 'NONE', #20500 ) ;
#20865=DIRECTION ( 'NONE',  ( -0.7313537016191752338, 0.6819983600624933695, 1.628001950178161200E-16 ) ) ;
#20871=CIRCLE ( 'NONE', #10711, 6.500000000000067502 ) ;
#20872=FACE_OUTER_BOUND ( 'NONE', #4750, .T. ) ;
#20873=CARTESIAN_POINT ( 'NONE',  ( 119.5756419024614132, 0.5000000000000004441, -6.499999999999964473 ) ) ;
#20880=VERTEX_POINT ( 'NONE', #1822 ) ;
#20891=EDGE_CURVE ( 'NONE', #11432, #3321, #2525, .T. ) ;
#20899=DIRECTION ( 'NONE',  ( -1.000000000000000000, 0.000000000000000000, -3.717264591378832268E-16 ) ) ;
#20910=VECTOR ( 'NONE', #16202, 1000.000000000000000 ) ;
#20917=EDGE_CURVE ( 'NONE', #22529, #20860, #7406, .T. ) ;
#20921=VERTEX_POINT ( 'NONE', #4940 ) ;
#20927=CIRCLE ( 'NONE', #20552, 7.000000000000075495 ) ;
#20940=AXIS2_PLACEMENT_3D ( 'NONE', #6410, #1122, #11808 ) ;
#20942=ORIENTED_EDGE ( 'NONE', *, *, #13844, .T. ) ;
#20955=DIRECTION ( 'NONE',  ( 1.000000000000000000, 2.699383410053119644E-30, 3.330669073875432643E-16 ) ) ;
#20959=LINE ( 'NONE', #22841, #2899 ) ;
#20963=CIRCLE ( 'NONE', #678, 6.500000000000075495 ) ;
#20964=ORIENTED_EDGE ( 'NONE', *, *, #19177, .F. ) ;
#20970=ORIENTED_EDGE ( 'NONE', *, *, #5079, .F. ) ;
#20973=CYLINDRICAL_SURFACE ( 'NONE', #13278, 7.000000000000075495 ) ;
#21001=AXIS2_PLACEMENT_3D ( 'NONE', #21711, #14871, #11326 ) ;
#21008=EDGE_CURVE ( 'NONE', #19367, #8320, #20959, .T. ) ;
#21011=DIRECTION ( 'NONE',  ( -1.000000000000000000, -2.699383410053119644E-30, -3.330669073875432643E-16 ) ) ;
#21015=DIRECTION ( 'NONE',  ( -0.7313537016191733464, 0.6819983600624954789, -3.733258675956564523E-18 ) ) ;
#21034=CYLINDRICAL_SURFACE ( 'NONE', #3159, 2.550000000000012701 ) ;
#21084=ORIENTED_EDGE ( 'NONE', *, *, #10734, .F. ) ;
#21085=ORIENTED_EDGE ( 'NONE', *, *, #11782, .F. ) ;
#21091=CARTESIAN_POINT ( 'NONE',  ( 86.00000000000122213, -10.52760560296347947, -5.999999999999998224 ) ) ;
#21094=CARTESIAN_POINT ( 'NONE',  ( 77.42435809754135789, -4.499999999999809930, 6.500000000000137668 ) ) ;
#21106=DIRECTION ( 'NONE',  ( -1.000000000000000000, 0.000000000000000000, -4.336808689941968432E-16 ) ) ;
#21111=EDGE_LOOP ( 'NONE', ( #22154, #12500, #23088, #1378 ) ) ;
#21117=ADVANCED_FACE ( 'NONE', ( #16683 ), #2576, .T. ) ;
#21127=CARTESIAN_POINT ( 'NONE',  ( 124.5000000000018616, -6.500000000000005329, 6.500000000000179412 ) ) ;
#21141=ORIENTED_EDGE ( 'NONE', *, *, #1086, .F. ) ;
#21152=DIRECTION ( 'NONE',  ( -0.6819983600625074693, 0.7313537016191621332, -1.110084618464482116E-16 ) ) ;
#21162=DIRECTION ( 'NONE',  ( 3.885780586188016830E-16, 4.437342591868156373E-31, -1.000000000000000000 ) ) ;
#21169=LINE ( 'NONE', #7903, #20186 ) ;
#21174=VECTOR ( 'NONE', #20231, 1000.000000000000114 ) ;
#21182=CARTESIAN_POINT ( 'NONE',  ( 77.42435809754137210, -6.499999999999811706, -5.999999999999984901 ) ) ;
#21184=LINE ( 'NONE', #5290, #12630 ) ;
#21216=ADVANCED_FACE ( 'NONE', ( #8109 ), #7992, .F. ) ;
#21230=DIRECTION ( 'NONE',  ( 3.885780586188016830E-16, 4.437342591868156373E-31, -1.000000000000000000 ) ) ;
#21249=FACE_OUTER_BOUND ( 'NONE', #15042, .T. ) ;
#21252=DIRECTION ( 'NONE',  ( -3.885780586188016830E-16, -4.437342591868156373E-31, 1.000000000000000000 ) ) ;
#21261=CARTESIAN_POINT ( 'NONE',  ( 66.26395429947835680, -6.500000000000005329, -6.500000000000081712 ) ) ;
#21267=ORIENTED_EDGE ( 'NONE', *, *, #2040, .F. ) ;
#21279=CARTESIAN_POINT ( 'NONE',  ( 63.53596085922838199, -4.500000000000059508, -6.000000000000060396 ) ) ;
#21284=DIRECTION ( 'NONE',  ( -3.885780586188016830E-16, -4.437342591868156373E-31, 1.000000000000000000 ) ) ;
#21321=ORIENTED_EDGE ( 'NONE', *, *, #14053, .T. ) ;
#21326=ORIENTED_EDGE ( 'NONE', *, *, #14111, .F. ) ;
#21339=EDGE_CURVE ( 'NONE', #7176, #13355, #5037, .T. ) ;
#21347=DIRECTION ( 'NONE',  ( -5.598259082250514647E-17, 1.000000000000000000, -6.162975822039315660E-32 ) ) ;
#21370=CARTESIAN_POINT ( 'NONE',  ( 63.50658097017377912, -4.000000000000003553, 6.500000000000151879 ) ) ;
#21373=CARTESIAN_POINT ( 'NONE',  ( 81.85734743794773749, -6.246200939475199831, 6.500000000000130562 ) ) ;
#21376=CARTESIAN_POINT ( 'NONE',  ( 57.49335071782236639, -0.7089083427137543580, 6.000000000000143885 ) ) ;
#21388=ORIENTED_EDGE ( 'NONE', *, *, #2806, .T. ) ;
#21391=ORIENTED_EDGE ( 'NONE', *, *, #9946, .F. ) ;
#21406=CARTESIAN_POINT ( 'NONE',  ( 116.5066492821802768, -7.708908342713760575, 6.500000000000151879 ) ) ;
#21410=EDGE_CURVE ( 'NONE', #6978, #16151, #14901, .T. ) ;
#21412=PLANE ( 'NONE',  #13433 ) ;
#21413=EDGE_LOOP ( 'NONE', ( #7680, #21651, #9243, #6642 ) ) ;
#21415=AXIS2_PLACEMENT_3D ( 'NONE', #10498, #12726, #2015 ) ;
#21418=ORIENTED_EDGE ( 'NONE', *, *, #4458, .F. ) ;
#21440=ORIENTED_EDGE ( 'NONE', *, *, #519, .T. ) ;
#21456=ADVANCED_FACE ( 'NONE', ( #5978 ), #11502, .T. ) ;
#21464=DIRECTION ( 'NONE',  ( -3.330669073875432643E-16, -4.437342591868153746E-31, 1.000000000000000000 ) ) ;
#21466=AXIS2_PLACEMENT_3D ( 'NONE', #3192, #15639, #22832 ) ;
#21471=EDGE_CURVE ( 'NONE', #8320, #16118, #3995, .T. ) ;
#21474=ORIENTED_EDGE ( 'NONE', *, *, #8981, .F. ) ;
#21475=EDGE_LOOP ( 'NONE', ( #2274, #16325, #7346, #18734 ) ) ;
#21486=AXIS2_PLACEMENT_3D ( 'NONE', #2481, #13432, #22134 ) ;
#21500=EDGE_CURVE ( 'NONE', #16775, #5606, #20799, .T. ) ;
#21512=DIRECTION ( 'NONE',  ( -4.336808689941983223E-16, 0.000000000000000000, 1.000000000000000000 ) ) ;
#21516=DIRECTION ( 'NONE',  ( -3.330669073875432643E-16, -4.437342591868153746E-31, 1.000000000000000000 ) ) ;
#21529=CIRCLE ( 'NONE', #22645, 0.5000000000000038858 ) ;
#21534=FACE_OUTER_BOUND ( 'NONE', #12598, .T. ) ;
#21537=CARTESIAN_POINT ( 'NONE',  ( 124.5000000000019043, -6.500000000000005329, 6.000000000000165201 ) ) ;
#21544=CARTESIAN_POINT ( 'NONE',  ( 88.75737332930593482, -6.527605602963476805, -6.499999999999929834 ) ) ;
#21549=CARTESIAN_POINT ( 'NONE',  ( 119.5756419024615553, -11.00000000000006573, 6.500000000000012434 ) ) ;
#21556=ORIENTED_EDGE ( 'NONE', *, *, #7052, .F. ) ;
#21563=CIRCLE ( 'NONE', #18539, 0.5000000000000038858 ) ;
#21565=DIRECTION ( 'NONE',  ( -3.885780586188016830E-16, -4.437342591868156373E-31, 1.000000000000000000 ) ) ;
#21576=DIRECTION ( 'NONE',  ( -0.7313537016191778983, -0.6819983600624907050, -2.183113462490731581E-16 ) ) ;
#21592=ORIENTED_EDGE ( 'NONE', *, *, #12844, .T. ) ;
#21606=CARTESIAN_POINT ( 'NONE',  ( 66.26395429947837101, 0.000000000000000000, -5.999999999999908518 ) ) ;
#21610=ORIENTED_EDGE ( 'NONE', *, *, #13244, .F. ) ;
#21618=VERTEX_POINT ( 'NONE', #21261 ) ;
#21619=ADVANCED_FACE ( 'NONE', ( #17954 ), #2490, .T. ) ;
#21623=LINE ( 'NONE', #17611, #8522 ) ;
#21627=DIRECTION ( 'NONE',  ( -1.000000000000000000, 1.847414967615758933E-47, -3.885780586188017323E-16 ) ) ;
#21628=DIRECTION ( 'NONE',  ( 0.7313537016191733464, -0.6819983600624954789, 3.733258675956564523E-18 ) ) ;
#21642=ADVANCED_FACE ( 'NONE', ( #5126 ), #6900, .T. ) ;
#21650=DIRECTION ( 'NONE',  ( 3.885780586188016830E-16, 4.437342591868156373E-31, -1.000000000000000000 ) ) ;
#21651=ORIENTED_EDGE ( 'NONE', *, *, #13844, .F. ) ;
#21671=ORIENTED_EDGE ( 'NONE', *, *, #1723, .T. ) ;
#21688=DIRECTION ( 'NONE',  ( -3.885780586188016830E-16, -4.437342591868156373E-31, 1.000000000000000000 ) ) ;
#21690=DIRECTION ( 'NONE',  ( 3.032184104443272185E-30, 1.000000000000000000, -7.395570986447005381E-32 ) ) ;
#21696=VERTEX_POINT ( 'NONE', #15936 ) ;
#21709=VECTOR ( 'NONE', #5100, 1000.000000000000000 ) ;
#21711=CARTESIAN_POINT ( 'NONE',  ( 112.6756160111034006, -11.28140466348826010, 6.000000000000032863 ) ) ;
#21714=CARTESIAN_POINT ( 'NONE',  ( 119.5756419024615269, -4.000000000000058620, -5.999999999999984901 ) ) ;
#21721=CARTESIAN_POINT ( 'NONE',  ( 108.2426266706970637, -6.527605602963671316, -5.999999999999991118 ) ) ;
#21746=CARTESIAN_POINT ( 'NONE',  ( 124.5000000000017195, -4.000000000000058620, 1.387778780781445676E-14 ) ) ;
#21752=EDGE_LOOP ( 'NONE', ( #21440, #10885, #21592, #2766 ) ) ;
#21761=DIRECTION ( 'NONE',  ( 3.885780586188016830E-16, 4.437342591868156373E-31, -1.000000000000000000 ) ) ;
#21764=DIRECTION ( 'NONE',  ( 0.000000000000000000, 0.000000000000000000, 1.000000000000000000 ) ) ;
#21765=CARTESIAN_POINT ( 'NONE',  ( 54.42435809754106657, -4.000000000000003553, 6.000000000000136779 ) ) ;
#21772=CARTESIAN_POINT ( 'NONE',  ( 56.00000000000088107, 0.000000000000000000, 6.500000000000117240 ) ) ;
#21774=CARTESIAN_POINT ( 'NONE',  ( 114.8016533820239005, -4.500000000000059508, -5.999999999999984901 ) ) ;
#21776=AXIS2_PLACEMENT_3D ( 'NONE', #9591, #12883, #542 ) ;
#21787=VERTEX_POINT ( 'NONE', #11332 ) ;
#21798=CARTESIAN_POINT ( 'NONE',  ( 108.2426266706970353, -13.52760560296359316, -6.000000000000019540 ) ) ;
#21816=LINE ( 'NONE', #18275, #20402 ) ;
#21833=DIRECTION ( 'NONE',  ( -1.000000000000000000, -2.699383410053119644E-30, -3.330669073875432643E-16 ) ) ;
#21840=CIRCLE ( 'NONE', #802, 2.550000000000024691 ) ;
#21841=TOROIDAL_SURFACE ( 'NONE', #15445, 6.000000000000015987, 0.5000000000000000000 ) ;
#21845=LINE ( 'NONE', #16524, #345 ) ;
#21847=CARTESIAN_POINT ( 'NONE',  ( 61.83096495907209089, -4.753799060524588782, 6.500000000000179412 ) ) ;
#21848=DIRECTION ( 'NONE',  ( 3.885780586188016830E-16, 4.437342591868156373E-31, -1.000000000000000000 ) ) ;
#21868=CARTESIAN_POINT ( 'NONE',  ( 86.00000000000133582, -13.02760560296348302, -5.999999999999956479 ) ) ;
#21871=AXIS2_PLACEMENT_3D ( 'NONE', #15930, #14949, #16580 ) ;
#21883=PRODUCT_CONTEXT ( 'NONE', #2628, 'mechanical' ) ;
#21898=CARTESIAN_POINT ( 'NONE',  ( 88.75737332930596324, -13.52760560296348302, -6.499999999999964473 ) ) ;
#21913=DIRECTION ( 'NONE',  ( 1.000000000000000000, 0.000000000000000000, 2.668805347656595124E-16 ) ) ;
#21914=EDGE_CURVE ( 'NONE', #4310, #7880, #4773, .T. ) ;
#21916=DIRECTION ( 'NONE',  ( -1.000000000000000000, -5.598259082250514647E-17, -3.330669073875432643E-16 ) ) ;
#21922=EDGE_CURVE ( 'NONE', #10566, #522, #2992, .T. ) ;
#21932=LINE ( 'NONE', #18623, #1621 ) ;
#21935=ORIENTED_EDGE ( 'NONE', *, *, #8723, .T. ) ;
#21936=AXIS2_PLACEMENT_3D ( 'NONE', #16546, #5872, #9507 ) ;
#21937=ORIENTED_EDGE ( 'NONE', *, *, #1912, .T. ) ;
#21944=DIRECTION ( 'NONE',  ( -1.000000000000000000, 4.780126911580487002E-14, -3.854941057726199147E-16 ) ) ;
#21954=VERTEX_POINT ( 'NONE', #14042 ) ;
#21958=ORIENTED_EDGE ( 'NONE', *, *, #23195, .F. ) ;
#21960=CYLINDRICAL_SURFACE ( 'NONE', #9165, 0.5000000000000026645 ) ;
#21975=( NAMED_UNIT ( * ) PLANE_ANGLE_UNIT ( ) SI_UNIT ( $, .RADIAN. ) );
#21982=DIRECTION ( 'NONE',  ( -0.7313537016191746787, -0.6819983600624941467, -1.072890437865584409E-16 ) ) ;
#21989=VECTOR ( 'NONE', #21761, 1000.000000000000000 ) ;
#21990=DIRECTION ( 'NONE',  ( 1.000000000000000000, -7.477632011778292156E-48, 3.885780586188017323E-16 ) ) ;
#21992=DIRECTION ( 'NONE',  ( -1.000000000000000000, -2.699383410053119644E-30, -3.330669073875432643E-16 ) ) ;
#21993=DIRECTION ( 'NONE',  ( 0.7313537016191746787, 0.6819983600624940356, 1.072890437865584409E-16 ) ) ;
#21998=FACE_OUTER_BOUND ( 'NONE', #277, .T. ) ;
#22008=ADVANCED_FACE ( 'NONE', ( #3108 ), #1568, .T. ) ;
#22019=EDGE_CURVE ( 'NONE', #273, #1495, #265, .T. ) ;
#22021=EDGE_CURVE ( 'NONE', #10139, #20178, #10508, .T. ) ;
#22046=DIRECTION ( 'NONE',  ( -0.6819983600625060260, -0.7313537016191634654, 0.000000000000000000 ) ) ;
#22058=ORIENTED_EDGE ( 'NONE', *, *, #11092, .F. ) ;
#22063=EDGE_LOOP ( 'NONE', ( #13925, #9618, #5693, #3884 ) ) ;
#22065=ORIENTED_EDGE ( 'NONE', *, *, #18864, .F. ) ;
#22067=EDGE_LOOP ( 'NONE', ( #13705, #22065, #23118, #4431 ) ) ;
#22069=DIRECTION ( 'NONE',  ( -1.000000000000000000, 1.696174065399527605E-14, -3.854941057726199147E-16 ) ) ;
#22075=CARTESIAN_POINT ( 'NONE',  ( 77.42435809754130105, -10.99999999999981526, 6.000000000000123457 ) ) ;
#22095=DIRECTION ( 'NONE',  ( 0.6819983600624951459, 0.7313537016191735685, 7.771699578536686021E-16 ) ) ;
#22104=TOROIDAL_SURFACE ( 'NONE', #11948, 4.500000000000000888, 0.5000000000000000000 ) ;
#22106=LINE ( 'NONE', #6344, #14691 ) ;
#22108=DIRECTION ( 'NONE',  ( 3.241725282392603095E-30, 1.000000000000000000, -2.218671295934100958E-31 ) ) ;
#22115=AXIS2_PLACEMENT_3D ( 'NONE', #4943, #2963, #5306 ) ;
#22117=AXIS2_PLACEMENT_3D ( 'NONE', #3514, #14328, #19751 ) ;
#22120=EDGE_CURVE ( 'NONE', #8376, #7460, #21169, .T. ) ;
#22127=FACE_OUTER_BOUND ( 'NONE', #3997, .T. ) ;
#22128=FACE_OUTER_BOUND ( 'NONE', #16770, .T. ) ;
#22134=DIRECTION ( 'NONE',  ( 0.000000000000000000, 0.000000000000000000, 1.000000000000000000 ) ) ;
#22138=CARTESIAN_POINT ( 'NONE',  ( 118.6341267379645501, -2.990348597579822965, 6.500000000000130562 ) ) ;
#22141=EDGE_LOOP ( 'NONE', ( #87, #10663, #10969, #6634 ) ) ;
#22154=ORIENTED_EDGE ( 'NONE', *, *, #10387, .T. ) ;
#22160=DIRECTION ( 'NONE',  ( -3.330669073875432643E-16, -4.437342591868153746E-31, 1.000000000000000000 ) ) ;
#22167=LINE ( 'NONE', #10984, #17220 ) ;
#22172=CARTESIAN_POINT ( 'NONE',  ( 108.2426266706970637, -10.52760560296347947, 6.500000000000019540 ) ) ;
#22176=CIRCLE ( 'NONE', #19914, 2.550000000000012701 ) ;
#22177=ORIENTED_EDGE ( 'NONE', *, *, #9946, .T. ) ;
#22180=EDGE_CURVE ( 'NONE', #12208, #10144, #15303, .T. ) ;
#22187=DIRECTION ( 'NONE',  ( -0.7313537016191756779, 0.6819983600624930364, -4.000536147326505450E-15 ) ) ;
#22191=DIRECTION ( 'NONE',  ( 0.7313537016191745677, 0.6819983600624940356, 1.072890437865584285E-16 ) ) ;
#22203=( LENGTH_UNIT ( ) NAMED_UNIT ( * ) SI_UNIT ( .MILLI., .METRE. ) );
#22207=ORIENTED_EDGE ( 'NONE', *, *, #17411, .F. ) ;
#22211=ORIENTED_EDGE ( 'NONE', *, *, #5015, .F. ) ;
#22216=EDGE_CURVE ( 'NONE', #5349, #22506, #17061, .T. ) ;
#22230=DIRECTION ( 'NONE',  ( 0.000000000000000000, 0.000000000000000000, -1.000000000000000000 ) ) ;
#22233=ORIENTED_EDGE ( 'NONE', *, *, #18416, .F. ) ;
#22238=LINE ( 'NONE', #16693, #17800 ) ;
#22244=CARTESIAN_POINT ( 'NONE',  ( 119.5756419024615411, -7.000000000000006217, 6.500000000000103029 ) ) ;
#22257=AXIS2_PLACEMENT_3D ( 'NONE', #4654, #8428, #13486 ) ;
#22263=EDGE_LOOP ( 'NONE', ( #13265, #3804, #2910, #10515 ) ) ;
#22265=ORIENTED_EDGE ( 'NONE', *, *, #2965, .T. ) ;
#22278=AXIS2_PLACEMENT_3D ( 'NONE', #7461, #3271, #10547 ) ;
#22285=FACE_OUTER_BOUND ( 'NONE', #19423, .T. ) ;
#22293=EDGE_LOOP ( 'NONE', ( #9427, #13264, #3019, #14135 ) ) ;
#22297=AXIS2_PLACEMENT_3D ( 'NONE', #375, #3885, #2004 ) ;
#22306=ORIENTED_EDGE ( 'NONE', *, *, #108, .T. ) ;
#22308=ADVANCED_FACE ( 'NONE', ( #3632, #17988 ), #21412, .F. ) ;
#22309=TOROIDAL_SURFACE ( 'NONE', #15161, 6.500000000000000888, 0.5000000000000000000 ) ;
#22312=DIRECTION ( 'NONE',  ( 3.885780586188016830E-16, 4.437342591868156373E-31, -1.000000000000000000 ) ) ;
#22315=CIRCLE ( 'NONE', #12155, 4.500000000000045297 ) ;
#22326=ORIENTED_EDGE ( 'NONE', *, *, #7529, .F. ) ;
#22363=AXIS2_PLACEMENT_3D ( 'NONE', #15774, #10491, #17660 ) ;
#22392=CARTESIAN_POINT ( 'NONE',  ( 88.75737332930594903, -6.527605602963476805, 6.500000000000151879 ) ) ;
#22411=ORIENTED_EDGE ( 'NONE', *, *, #1271, .T. ) ;
#22423=DIRECTION ( 'NONE',  ( 0.6819983600624957010, 0.7313537016191731244, 7.771699578536735325E-16 ) ) ;
#22429=DIRECTION ( 'NONE',  ( 0.7313537016191746787, 0.6819983600624940356, 1.072890437865584409E-16 ) ) ;
#22446=CARTESIAN_POINT ( 'NONE',  ( 88.75737332930586376, -10.52760560296347947, 6.000000000000165201 ) ) ;
#22455=DIRECTION ( 'NONE',  ( 3.032184104443271834E-30, 1.000000000000000000, 4.437342591868167759E-31 ) ) ;
#22457=DIRECTION ( 'NONE',  ( 1.000000000000000000, 2.699383410053119644E-30, 3.330669073875432643E-16 ) ) ;
#22467=AXIS2_PLACEMENT_3D ( 'NONE', #15819, #23018, #5131 ) ;
#22491=AXIS2_PLACEMENT_3D ( 'NONE', #2435, #16889, #20214 ) ;
#22497=EDGE_LOOP ( 'NONE', ( #7719, #3238, #21267, #21935 ) ) ;
#22506=VERTEX_POINT ( 'NONE', #6561 ) ;
#22516=DIRECTION ( 'NONE',  ( -1.000000000000000000, -2.699383410053119644E-30, -3.330669073875432643E-16 ) ) ;
#22519=FACE_OUTER_BOUND ( 'NONE', #1211, .T. ) ;
#22528=ORIENTED_EDGE ( 'NONE', *, *, #15426, .T. ) ;
#22529=VERTEX_POINT ( 'NONE', #4545 ) ;
#22540=CARTESIAN_POINT ( 'NONE',  ( 108.9540049198142242, -11.33354449810611264, -6.000000000000074607 ) ) ;
#22561=CARTESIAN_POINT ( 'NONE',  ( 119.5756419024615269, -11.00000000000006573, 6.000000000000081712 ) ) ;
#22568=FACE_OUTER_BOUND ( 'NONE', #11374, .T. ) ;
#22575=DIRECTION ( 'NONE',  ( 0.000000000000000000, 0.000000000000000000, 1.000000000000000000 ) ) ;
#22582=ORIENTED_EDGE ( 'NONE', *, *, #15592, .T. ) ;
#22591=FACE_OUTER_BOUND ( 'NONE', #21111, .T. ) ;
#22593=DIRECTION ( 'NONE',  ( -1.000000000000000000, -2.699383410053119644E-30, -3.330669073875432643E-16 ) ) ;
#22601=FACE_OUTER_BOUND ( 'NONE', #9012, .T. ) ;
#22610=VERTEX_POINT ( 'NONE', #17355 ) ;
#22617=DIRECTION ( 'NONE',  ( -3.885780586188016830E-16, -4.437342591868156373E-31, 1.000000000000000000 ) ) ;
#22621=ADVANCED_FACE ( 'NONE', ( #22787 ), #4426, .T. ) ;
#22630=CARTESIAN_POINT ( 'NONE',  ( 6.500000000000339284, 2.500000000000141220, -6.499999999999950262 ) ) ;
#22639=EDGE_CURVE ( 'NONE', #8580, #9470, #20207, .T. ) ;
#22640=ORIENTED_EDGE ( 'NONE', *, *, #6444, .F. ) ;
#22644=ORIENTED_EDGE ( 'NONE', *, *, #18747, .T. ) ;
#22645=AXIS2_PLACEMENT_3D ( 'NONE', #1929, #12406, #2165 ) ;
#22649=AXIS2_PLACEMENT_3D ( 'NONE', #9005, #21252, #5118 ) ;
#22653=ADVANCED_BREP_SHAPE_REPRESENTATION ( '', ( #20836, #22115 ), #712 ) ;
#22657=DIRECTION ( 'NONE',  ( -0.7313537016191746787, -0.6819983600624940356, -1.072890437865584409E-16 ) ) ;
#22661=DIRECTION ( 'NONE',  ( 3.885780586188016830E-16, 4.437342591868156373E-31, -1.000000000000000000 ) ) ;
#22664=AXIS2_PLACEMENT_3D ( 'NONE', #10180, #17346, #15810 ) ;
#22673=CIRCLE ( 'NONE', #17000, 7.000000000000089706 ) ;
#22680=VERTEX_POINT ( 'NONE', #19365 ) ;
#22683=CARTESIAN_POINT ( 'NONE',  ( 111.3116192909783422, -9.818697260249892977, 6.500000000000012434 ) ) ;
#22689=AXIS2_PLACEMENT_3D ( 'NONE', #17397, #8477, #22830 ) ;
#22692=VECTOR ( 'NONE', #19171, 1000.000000000000000 ) ;
#22696=CARTESIAN_POINT ( 'NONE',  ( 88.75737332930597745, -13.02760560296348302, -6.000000000000039968 ) ) ;
#22700=DIRECTION ( 'NONE',  ( 0.000000000000000000, 0.000000000000000000, 1.000000000000000000 ) ) ;
#22718=DIRECTION ( 'NONE',  ( 0.7313537016191735685, -0.6819983600624951459, 3.923113172947598083E-16 ) ) ;
#22725=EDGE_CURVE ( 'NONE', #4606, #12089, #8549, .T. ) ;
#22746=EDGE_CURVE ( 'NONE', #7130, #9737, #3315, .T. ) ;
#22749=ADVANCED_FACE ( 'NONE', ( #3263 ), #8662, .T. ) ;
#22759=ORIENTED_EDGE ( 'NONE', *, *, #13478, .T. ) ;
#22766=CYLINDRICAL_SURFACE ( 'NONE', #16663, 0.4999999999999987232 ) ;
#22769=EDGE_CURVE ( 'NONE', #7130, #4606, #19453, .T. ) ;
#22774=ADVANCED_FACE ( 'NONE', ( #1231 ), #2639, .T. ) ;
#22779=EDGE_CURVE ( 'NONE', #16059, #16601, #18992, .T. ) ;
#22782=AXIS2_PLACEMENT_3D ( 'NONE', #8308, #1254, #13721 ) ;
#22785=EDGE_LOOP ( 'NONE', ( #1096, #7343, #7695, #11712 ) ) ;
#22787=FACE_OUTER_BOUND ( 'NONE', #12235, .T. ) ;
#22794=EDGE_LOOP ( 'NONE', ( #1427, #16465, #17040, #17606 ) ) ;
#22796=ORIENTED_EDGE ( 'NONE', *, *, #4507, .T. ) ;
#22808=VECTOR ( 'NONE', #4594, 1000.000000000000000 ) ;
#22810=CARTESIAN_POINT ( 'NONE',  ( 118.0000000000018190, -6.500000000000061284, -6.000000000000012434 ) ) ;
#22812=CIRCLE ( 'NONE', #10388, 6.500000000000075495 ) ;
#22816=ORIENTED_EDGE ( 'NONE', *, *, #20439, .F. ) ;
#22825=ORIENTED_EDGE ( 'NONE', *, *, #8652, .F. ) ;
#22826=CARTESIAN_POINT ( 'NONE',  ( 108.2426266706970353, -10.52760560296359138, -6.000000000000019540 ) ) ;
#22830=DIRECTION ( 'NONE',  ( 0.000000000000000000, 0.000000000000000000, 1.000000000000000000 ) ) ;
#22832=DIRECTION ( 'NONE',  ( -4.003208021484906984E-16, 7.395570986447125806E-32, 1.000000000000000000 ) ) ;
#22841=CARTESIAN_POINT ( 'NONE',  ( 124.5000000000018900, -13.52760560296373171, 6.500000000000068390 ) ) ;
#22843=CARTESIAN_POINT ( 'NONE',  ( 6.500000000000227374, 3.000000000000169198, 4.163336342344337027E-14 ) ) ;
#22844=AXIS2_PLACEMENT_3D ( 'NONE', #18453, #9630, #20462 ) ;
#22863=DIRECTION ( 'NONE',  ( -1.000000000000000000, -2.699383410053119293E-30, -4.336808689941968432E-16 ) ) ;
#22876=ORIENTED_EDGE ( 'NONE', *, *, #12201, .F. ) ;
#22897=DIRECTION ( 'NONE',  ( -3.885780586188016830E-16, -4.437342591868156373E-31, 1.000000000000000000 ) ) ;
#22899=CYLINDRICAL_SURFACE ( 'NONE', #1909, 0.5000000000000038858 ) ;
#22908=CIRCLE ( 'NONE', #11255, 4.000000000000045297 ) ;
#22914=EDGE_CURVE ( 'NONE', #21618, #13307, #16809, .T. ) ;
#22920=DIRECTION ( 'NONE',  ( -5.598259082250079541E-17, 1.000000000000000000, -6.162975822039171151E-32 ) ) ;
#22924=AXIS2_PLACEMENT_3D ( 'NONE', #16957, #18853, #2737 ) ;
#22930=ADVANCED_FACE ( 'NONE', ( #4858 ), #13918, .F. ) ;
#22933=LINE ( 'NONE', #3730, #18308 ) ;
#22968=ORIENTED_EDGE ( 'NONE', *, *, #14775, .F. ) ;
#22979=CARTESIAN_POINT ( 'NONE',  ( 119.5756419024615838, -11.00000000000006573, -6.500000000000075495 ) ) ;
#22992=ORIENTED_EDGE ( 'NONE', *, *, #2937, .F. ) ;
#23000=AXIS2_PLACEMENT_3D ( 'NONE', #15727, #15492, #12190 ) ;
#23002=ORIENTED_EDGE ( 'NONE', *, *, #18416, .T. ) ;
#23007=DIRECTION ( 'NONE',  ( 1.000000000000000000, 2.699383410053119644E-30, 3.330669073875432643E-16 ) ) ;
#23009=FACE_OUTER_BOUND ( 'NONE', #16717, .T. ) ;
#23018=DIRECTION ( 'NONE',  ( 3.330669073875432643E-16, 4.437342591868153746E-31, -1.000000000000000000 ) ) ;
#23051=FACE_OUTER_BOUND ( 'NONE', #12353, .T. ) ;
#23053=ORIENTED_EDGE ( 'NONE', *, *, #15321, .F. ) ;
#23055=AXIS2_PLACEMENT_3D ( 'NONE', #3703, #1928, #14181 ) ;
#23073=CARTESIAN_POINT ( 'NONE',  ( 6.500000000000005329, -13.52760560296348302, -6.500000000000075495 ) ) ;
#23074=EDGE_CURVE ( 'NONE', #20880, #700, #11078, .T. ) ;
#23078=AXIS2_PLACEMENT_3D ( 'NONE', #4300, #13373, #15360 ) ;
#23079=DIRECTION ( 'NONE',  ( 1.000000000000000000, 2.699383410053119644E-30, 3.330669073875432643E-16 ) ) ;
#23088=ORIENTED_EDGE ( 'NONE', *, *, #17247, .F. ) ;
#23098=AXIS2_PLACEMENT_3D ( 'NONE', #12271, #8422, #12397 ) ;
#23100=FACE_OUTER_BOUND ( 'NONE', #15547, .T. ) ;
#23108=CARTESIAN_POINT ( 'NONE',  ( 81.04599508018874587, -4.805938895142302769, 6.000000000000116351 ) ) ;
#23116=DIRECTION ( 'NONE',  ( 1.000000000000000000, 2.699383410053119644E-30, 3.330669073875432643E-16 ) ) ;
#23117=VERTEX_POINT ( 'NONE', #2487 ) ;
#23118=ORIENTED_EDGE ( 'NONE', *, *, #13810, .F. ) ;
#23119=EDGE_LOOP ( 'NONE', ( #21321, #12983, #9879, #19193 ) ) ;
#23121=ORIENTED_EDGE ( 'NONE', *, *, #4458, .T. ) ;
#23126=TOROIDAL_SURFACE ( 'NONE', #3587, 6.000000000000015987, 0.5000000000000000000 ) ;
#23128=PLANE ( 'NONE',  #4613 ) ;
#23130=FACE_OUTER_BOUND ( 'NONE', #1667, .T. ) ;
#23134=DIRECTION ( 'NONE',  ( -3.885780586188016830E-16, -4.437342591868156373E-31, 1.000000000000000000 ) ) ;
#23147=ORIENTED_EDGE ( 'NONE', *, *, #19473, .F. ) ;
#23176=VERTEX_POINT ( 'NONE', #6147 ) ;
#23184=CARTESIAN_POINT ( 'NONE',  ( 114.8016533820240568, -5.880524088665878502, -6.499999999999970690 ) ) ;
#23186=ORIENTED_EDGE ( 'NONE', *, *, #11079, .T. ) ;
#23195=EDGE_CURVE ( 'NONE', #19862, #8293, #17178, .T. ) ;
#23206=ORIENTED_EDGE ( 'NONE', *, *, #22120, .T. ) ;
#23211=ORIENTED_EDGE ( 'NONE', *, *, #8790, .T. ) ;
#23214=DIRECTION ( 'NONE',  ( -3.885780586188016830E-16, -4.437342591868156373E-31, 1.000000000000000000 ) ) ;
#23219=CARTESIAN_POINT ( 'NONE',  ( 110.9706201109471522, -9.453020409440348715, 6.000000000000088818 ) ) ;
#23226=CARTESIAN_POINT ( 'NONE',  ( 119.5756419024615269, -4.500000000000059508, -5.999999999999984901 ) ) ;
#23228=CARTESIAN_POINT ( 'NONE',  ( 116.5066492821803195, -7.708908342713815642, -5.999999999999998224 ) ) ;
#23231=CARTESIAN_POINT ( 'NONE',  ( 63.50658097017372938, -7.000000000000006217, 6.500000000000068390 ) ) ;
#23252=CARTESIAN_POINT ( 'NONE',  ( 57.49335071782242323, -0.7089083427137543580, -6.499999999999922728 ) ) ;
#23253=CARTESIAN_POINT ( 'NONE',  ( 124.5000000000019185, -7.000000000000062172, -5.999999999999984901 ) ) ;
#23264=DIRECTION ( 'NONE',  ( 0.000000000000000000, 0.000000000000000000, 1.000000000000000000 ) ) ;
#23265=AXIS2_PLACEMENT_3D ( 'NONE', #14414, #6767, #13935 ) ;
#23267=ORIENTED_EDGE ( 'NONE', *, *, #6362, .T. ) ;
ENDSEC;
END-ISO-10303-21;
